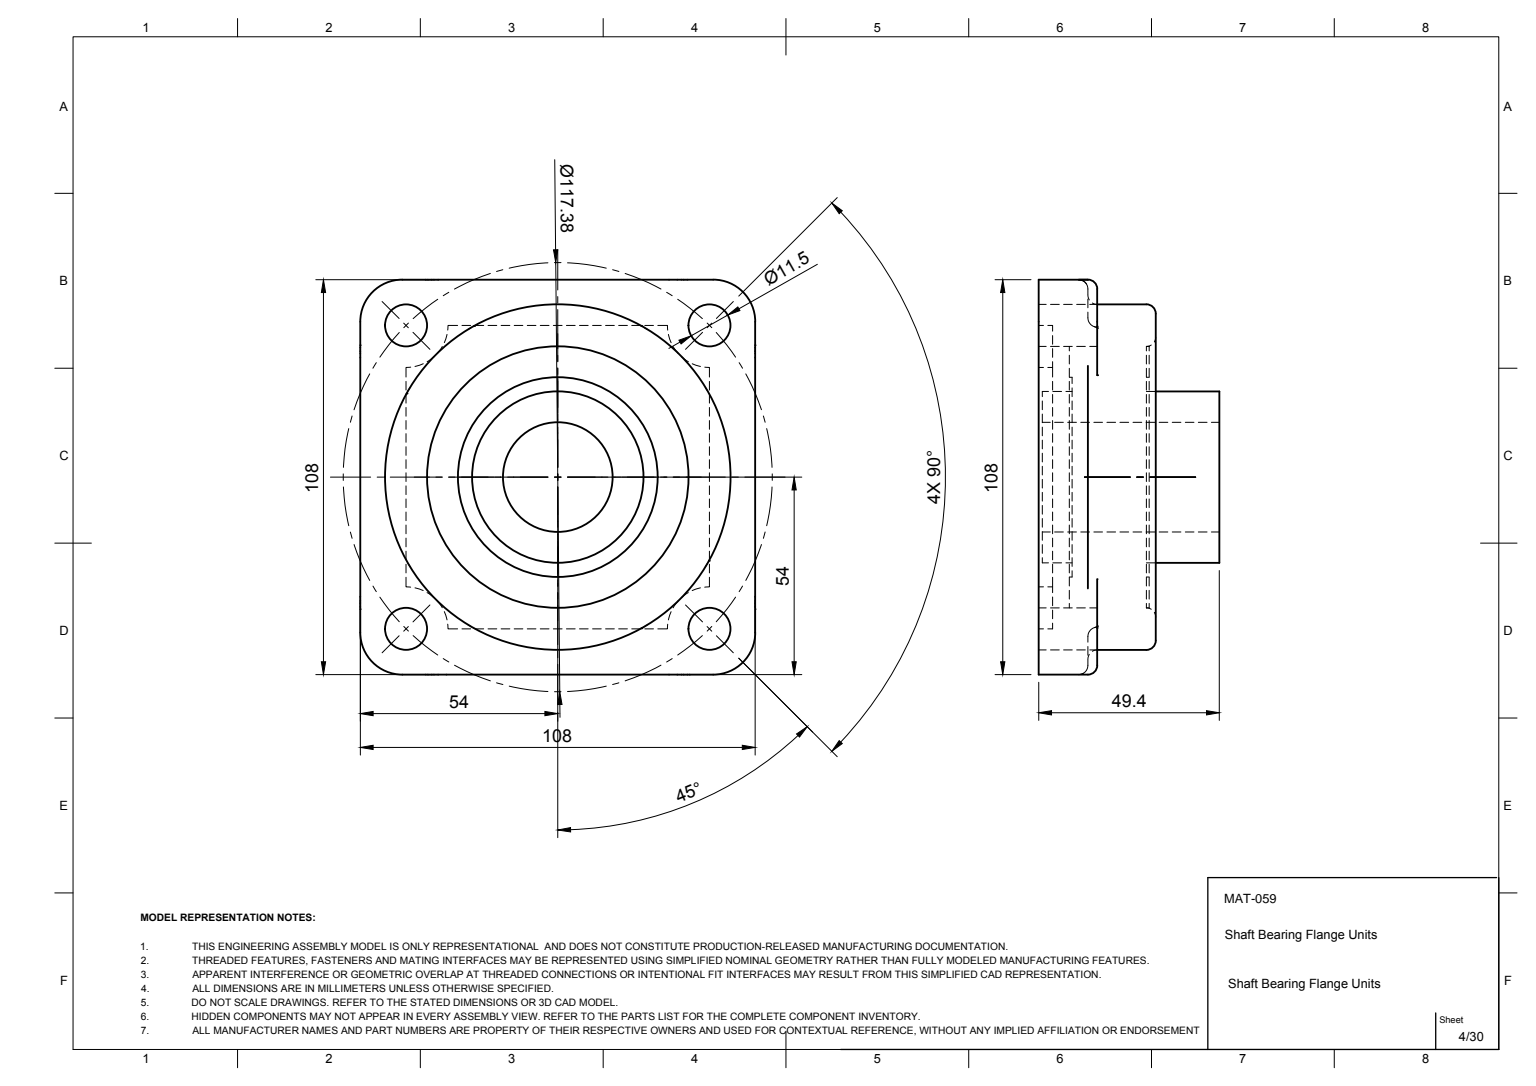
ISO-10303-21;
HEADER;
/* Generated by software containing ST-Developer
 * from STEP Tools, Inc. (www.steptools.com) 
 */

FILE_DESCRIPTION(
/* description */ ('', 'CAx-IF Rec.Pracs.---Representation and Presentation of Product Manufa
cturing Information (PMI)---4.0---2014-10-13'),
/* implementation_level */ '2;1');

FILE_NAME(
/* name */ 'Shaft Bearing Flange Units.step',
/* time_stamp */ '2026-10-28T23:00:48+01:00',
/* author */ (''),
/* organization */ (''),
/* preprocessor_version */ 'ST-DEVELOPER v20.2',
/* originating_system */ 'Autodesk Translation Framework v15.17.0.0',
/* authorisation */ '');

FILE_SCHEMA (('AP242_MANAGED_MODEL_BASED_3D_ENGINEERING_MIM_LF { 1 0 10303 442 2 1 4 }'));
ENDSEC;

DATA;
#10=MECHANICAL_DESIGN_GEOMETRIC_PRESENTATION_REPRESENTATION('',(#962),#61811);
#710=SPHERICAL_SURFACE('',#34223,2.54);
#711=SPHERICAL_SURFACE('',#34226,2.54);
#712=SPHERICAL_SURFACE('',#34247,2.54);
#713=SPHERICAL_SURFACE('',#34253,2.54);
#714=SPHERICAL_SURFACE('',#34261,2.54);
#715=SPHERICAL_SURFACE('',#34268,2.54);
#716=SPHERICAL_SURFACE('',#34273,2.54);
#717=SPHERICAL_SURFACE('',#34278,2.54);
#718=SPHERICAL_SURFACE('',#34289,2.54);
#719=SPHERICAL_SURFACE('',#34304,2.54);
#720=SPHERICAL_SURFACE('',#34315,2.54);
#721=SPHERICAL_SURFACE('',#34321,2.54);
#722=SPHERICAL_SURFACE('',#34322,2.54);
#723=SPHERICAL_SURFACE('',#34332,2.54);
#724=SPHERICAL_SURFACE('',#34340,2.54);
#725=SPHERICAL_SURFACE('',#34343,2.54);
#743=B_SPLINE_CURVE_WITH_KNOTS('',3,(#49121,#49122,#49123,#49124,#49125,
#49126,#49127,#49128,#49129),.UNSPECIFIED.,.F.,.F.,(4,1,1,1,1,1,4),(2.41610505192759E-5,
0.1666666666667,0.3333333333333,0.5,0.6666666666667,0.8333333333333,1.),
 .UNSPECIFIED.);
#744=B_SPLINE_CURVE_WITH_KNOTS('',3,(#49132,#49133,#49134,#49135,#49136,
#49137,#49138,#49139,#49140,#49141,#49142,#49143,#49144,#49145,#49146,#49147,
#49148,#49149,#49150,#49151,#49152,#49153),.UNSPECIFIED.,.F.,.F.,(4,2,2,
2,2,2,2,2,2,2,4),(0.,0.122614489199661,0.166666475605304,0.333332951210507,
0.341573133516598,0.499999426815811,0.560641811243984,0.666665902421115,
0.779351949400631,0.833332378026318,0.999998853631622),.UNSPECIFIED.);
#745=B_SPLINE_CURVE_WITH_KNOTS('',3,(#49162,#49163,#49164,#49165,#49166,
#49167,#49168,#49169,#49170),.UNSPECIFIED.,.F.,.F.,(4,1,1,1,1,1,4),(0.,
0.1666666666667,0.3333333333333,0.5,0.6666666666667,0.8333333333333,1.),
 .UNSPECIFIED.);
#746=B_SPLINE_CURVE_WITH_KNOTS('',3,(#49174,#49175,#49176,#49177,#49178,
#49179,#49180,#49181,#49182),.UNSPECIFIED.,.F.,.F.,(4,1,1,1,1,1,4),(2.85381265954449E-5,
0.1666666666667,0.3333333333333,0.5,0.6666666666667,0.8333333333333,1.),
 .UNSPECIFIED.);
#747=B_SPLINE_CURVE_WITH_KNOTS('',3,(#49186,#49187,#49188,#49189,#49190,
#49191,#49192,#49193,#49194),.UNSPECIFIED.,.F.,.F.,(4,1,1,1,1,1,4),(0.,
0.1666666666667,0.3333333333333,0.5,0.6666666666667,0.8333333333333,1.),
 .UNSPECIFIED.);
#748=B_SPLINE_CURVE_WITH_KNOTS('',3,(#49198,#49199,#49200,#49201,#49202,
#49203,#49204,#49205,#49206),.UNSPECIFIED.,.F.,.F.,(4,1,1,1,1,1,4),(2.416105051936E-5,
0.1666666666667,0.3333333333333,0.5,0.6666666666667,0.8333333333333,1.),
 .UNSPECIFIED.);
#749=B_SPLINE_CURVE_WITH_KNOTS('',3,(#49210,#49211,#49212,#49213,#49214,
#49215,#49216,#49217,#49218),.UNSPECIFIED.,.F.,.F.,(4,1,1,1,1,1,4),(0.,
0.1666666666667,0.3333333333333,0.5,0.6666666666667,0.8333333333333,1.),
 .UNSPECIFIED.);
#750=B_SPLINE_CURVE_WITH_KNOTS('',3,(#49222,#49223,#49224,#49225,#49226,
#49227,#49228,#49229,#49230),.UNSPECIFIED.,.F.,.F.,(4,1,1,1,1,1,4),(2.85380852244383E-5,
0.1666666666667,0.3333333333333,0.5,0.6666666666667,0.8333333333333,1.),
 .UNSPECIFIED.);
#751=B_SPLINE_CURVE_WITH_KNOTS('',3,(#49234,#49235,#49236,#49237,#49238,
#49239,#49240,#49241,#49242),.UNSPECIFIED.,.F.,.F.,(4,1,1,1,1,1,4),(0.,
0.1666666666667,0.3333333333333,0.5,0.6666666666667,0.8333333333333,0.999977439421937),
 .UNSPECIFIED.);
#752=B_SPLINE_CURVE_WITH_KNOTS('',3,(#49287,#49288,#49289,#49290,#49291,
#49292,#49293,#49294,#49295,#49296,#49297,#49298,#49299,#49300,#49301,#49302,
#49303,#49304,#49305,#49306,#49307,#49308,#49309,#49310,#49311,#49312,#49313,
#49314,#49315,#49316,#49317,#49318,#49319,#49320,#49321,#49322,#49323,#49324,
#49325,#49326,#49327,#49328,#49329,#49330,#49331,#49332,#49333,#49334,#49335,
#49336,#49337,#49338,#49339,#49340,#49341),.UNSPECIFIED.,.F.,.F.,(4,3,3,
3,3,3,3,3,3,3,3,3,3,3,3,3,3,3,4),(0.,0.0980466098756701,0.1428571428571,
0.235655762730469,0.2857142857143,0.360443887258383,0.4285714285714,0.5,
0.566042537085864,0.5714285714286,0.636887704333111,0.700301860505849,0.7142857142857,
0.779698786568794,0.844149904052703,0.8571428571429,0.915815433596542,0.97252549736179,
0.999999999993428),.UNSPECIFIED.);
#753=B_SPLINE_CURVE_WITH_KNOTS('',3,(#49366,#49367,#49368,#49369,#49370,
#49371,#49372,#49373,#49374,#49375),.UNSPECIFIED.,.F.,.F.,(4,1,1,1,1,1,
1,4),(0.,0.1428571428571,0.2857142857143,0.4285714285714,0.5714285714286,
0.7142857142857,0.8571428571429,1.),.UNSPECIFIED.);
#754=B_SPLINE_CURVE_WITH_KNOTS('',3,(#49379,#49380,#49381,#49382,#49383,
#49384,#49385,#49386,#49387,#49388),.UNSPECIFIED.,.F.,.F.,(4,1,1,1,1,1,
1,4),(0.,0.1428571428571,0.2857142857143,0.4285714285714,0.5714285714286,
0.7142857142857,0.8571428571429,1.),.UNSPECIFIED.);
#755=B_SPLINE_CURVE_WITH_KNOTS('',3,(#49403,#49404,#49405,#49406,#49407,
#49408,#49409,#49410,#49411,#49412),.UNSPECIFIED.,.F.,.F.,(4,1,1,1,1,1,
1,4),(0.,0.1428571428571,0.2857142857143,0.4285714285714,0.5714285714286,
0.7142857142857,0.8571428571429,1.),.UNSPECIFIED.);
#756=B_SPLINE_CURVE_WITH_KNOTS('',3,(#49415,#49416,#49417,#49418,#49419,
#49420,#49421,#49422,#49423,#49424),.UNSPECIFIED.,.F.,.F.,(4,1,1,1,1,1,
1,4),(0.,0.1428571428571,0.2857142857143,0.4285714285714,0.5714285714286,
0.7142857142857,0.8571428571429,1.),.UNSPECIFIED.);
#757=B_SPLINE_CURVE_WITH_KNOTS('',3,(#49471,#49472,#49473,#49474,#49475,
#49476,#49477,#49478,#49479,#49480,#49481,#49482,#49483,#49484,#49485,#49486,
#49487,#49488,#49489,#49490,#49491,#49492,#49493,#49494,#49495,#49496,#49497,
#49498,#49499,#49500,#49501,#49502,#49503,#49504,#49505,#49506,#49507,#49508,
#49509,#49510,#49511,#49512,#49513,#49514,#49515,#49516,#49517,#49518,#49519,
#49520,#49521,#49522,#49523,#49524,#49525,#49526,#49527,#49528,#49529,#49530,
#49531,#49532,#49533,#49534),.UNSPECIFIED.,.F.,.F.,(4,3,3,3,3,3,3,3,3,3,
3,3,3,3,3,3,3,3,3,3,3,4),(0.,0.022524348752069,0.0826907458045845,0.1428571428571,
0.183969209185199,0.24216625125188,0.2857142857143,0.344939441940217,0.408805968765505,
0.4285714285714,0.494637391748715,0.505902092667849,0.5714285714286,0.644329623937483,
0.666612808947293,0.7142857142857,0.786343515622748,0.827515831049201,0.8571428571429,
0.931638703404591,0.988736971542743,1.),.UNSPECIFIED.);
#758=B_SPLINE_CURVE_WITH_KNOTS('',3,(#49535,#49536,#49537,#49538,#49539,
#49540,#49541,#49542,#49543,#49544,#49545,#49546,#49547,#49548,#49549,#49550,
#49551,#49552,#49553,#49554,#49555,#49556,#49557,#49558,#49559,#49560,#49561,
#49562,#49563,#49564,#49565,#49566,#49567,#49568,#49569,#49570,#49571,#49572,
#49573,#49574,#49575,#49576,#49577),.UNSPECIFIED.,.F.,.F.,(4,3,3,3,3,3,
3,3,3,3,3,3,3,3,4),(0.,0.0708403169631036,0.141196221399192,0.211480985838496,
0.25,0.351421886552124,0.450884598470819,0.5,0.591484098710409,0.684303235352195,
0.75,0.824311643104987,0.900296423629433,0.978409207800814,0.999992340412632),
 .UNSPECIFIED.);
#759=B_SPLINE_CURVE_WITH_KNOTS('',3,(#49622,#49623,#49624,#49625,#49626,
#49627,#49628,#49629,#49630,#49631,#49632,#49633,#49634,#49635,#49636,#49637,
#49638,#49639,#49640,#49641,#49642,#49643),.UNSPECIFIED.,.F.,.F.,(4,2,2,
2,2,2,2,2,2,2,4),(1.17968190133454E-6,0.166667646133106,0.219922777256081,
0.333334116906424,0.439180276291458,0.500000587679843,0.658731994343029,
0.666667058453262,0.833333529226581,0.87820409141329,1.),.UNSPECIFIED.);
#760=B_SPLINE_CURVE_WITH_KNOTS('',3,(#49690,#49691,#49692,#49693,#49694,
#49695,#49696,#49697,#49698),.UNSPECIFIED.,.F.,.F.,(4,1,1,1,1,1,4),(0.,
0.1666666666667,0.3333333333333,0.5,0.6666666666667,0.8333333333333,0.999998808810884),
 .UNSPECIFIED.);
#761=B_SPLINE_CURVE_WITH_KNOTS('',3,(#49749,#49750,#49751,#49752,#49753,
#49754,#49755,#49756,#49757,#49758,#49759,#49760,#49761,#49762,#49763,#49764,
#49765,#49766,#49767,#49768,#49769,#49770,#49771,#49772,#49773,#49774,#49775,
#49776,#49777,#49778,#49779,#49780,#49781,#49782,#49783,#49784,#49785,#49786,
#49787,#49788,#49789,#49790,#49791,#49792,#49793,#49794,#49795,#49796,#49797,
#49798,#49799,#49800,#49801,#49802,#49803,#49804,#49805,#49806,#49807,#49808,
#49809,#49810,#49811,#49812),.UNSPECIFIED.,.F.,.F.,(4,3,3,3,3,3,3,3,3,3,
3,3,3,3,3,3,3,3,3,3,3,4),(0.,0.011263028288939,0.0857588259046287,0.1428571428571,
0.172484168893865,0.244542016262902,0.2857142857143,0.33338719123398,0.406288255376173,
0.4285714285714,0.49409790740126,0.560163866020983,0.5714285714286,0.635295097422919,
0.655060558117981,0.7142857142857,0.77248275702656,0.81603079085385,0.8571428571429,
0.917309254199729,0.977475651256559,1.),.UNSPECIFIED.);
#762=B_SPLINE_CURVE_WITH_KNOTS('',3,(#49861,#49862,#49863,#49864,#49865,
#49866,#49867,#49868,#49869,#49870,#49871,#49872,#49873,#49874,#49875,#49876,
#49877,#49878,#49879,#49880,#49881,#49882,#49883,#49884,#49885,#49886,#49887,
#49888,#49889,#49890,#49891,#49892,#49893,#49894,#49895,#49896,#49897,#49898,
#49899,#49900,#49901,#49902,#49903,#49904,#49905,#49906,#49907,#49908,#49909,
#49910,#49911,#49912,#49913,#49914,#49915,#49916,#49917,#49918,#49919,#49920,
#49921,#49922,#49923,#49924),.UNSPECIFIED.,.F.,.F.,(4,3,3,3,3,3,3,3,3,3,
3,3,3,3,3,3,3,3,3,3,3,4),(0.,0.022524348752069,0.0826907458045845,0.1428571428571,
0.183969209185192,0.242166251253732,0.2857142857143,0.34493944194013,0.408805968765661,
0.4285714285714,0.494637391744036,0.505902092667695,0.5714285714286,0.644329623939086,
0.666612808947312,0.7142857142857,0.786343515622548,0.827515831048836,0.8571428571429,
0.931638703405425,0.988736971542787,1.),.UNSPECIFIED.);
#763=B_SPLINE_CURVE_WITH_KNOTS('',3,(#49925,#49926,#49927,#49928,#49929,
#49930,#49931,#49932,#49933,#49934,#49935,#49936,#49937,#49938,#49939,#49940,
#49941,#49942,#49943,#49944,#49945,#49946,#49947,#49948,#49949,#49950,#49951,
#49952,#49953,#49954,#49955,#49956,#49957,#49958,#49959,#49960,#49961,#49962,
#49963,#49964,#49965,#49966,#49967),.UNSPECIFIED.,.F.,.F.,(4,3,3,3,3,3,
3,3,3,3,3,3,3,3,4),(0.,0.0708403169625752,0.141196221398188,0.211480985837894,
0.25,0.351421886557641,0.45088459847787,0.5,0.591484098711512,0.684303235350053,
0.75,0.824311643104386,0.900296423628743,0.978409207797605,0.999992340412643),
 .UNSPECIFIED.);
#764=B_SPLINE_CURVE_WITH_KNOTS('',3,(#50011,#50012,#50013,#50014,#50015,
#50016,#50017,#50018,#50019),.UNSPECIFIED.,.F.,.F.,(4,1,1,1,1,1,4),(1.12301924736311E-6,
0.1666666666667,0.3333333333333,0.5,0.6666666666667,0.8333333333333,1.),
 .UNSPECIFIED.);
#765=B_SPLINE_CURVE_WITH_KNOTS('',3,(#50069,#50070,#50071,#50072,#50073,
#50074,#50075,#50076,#50077,#50078,#50079,#50080,#50081,#50082,#50083,#50084,
#50085,#50086,#50087,#50088,#50089,#50090),.UNSPECIFIED.,.F.,.F.,(4,2,2,
2,2,2,2,2,2,2,4),(1.17968190350786E-6,0.166667646133105,0.219922777256189,
0.333334116906424,0.439180276291488,0.500000587679843,0.658731994343154,
0.666667058453262,0.833333529226581,0.878204091413217,1.),.UNSPECIFIED.);
#766=B_SPLINE_CURVE_WITH_KNOTS('',3,(#50099,#50100,#50101,#50102,#50103,
#50104,#50105,#50106,#50107,#50108,#50109,#50110,#50111,#50112,#50113,#50114,
#50115,#50116,#50117,#50118,#50119,#50120,#50121,#50122,#50123,#50124,#50125,
#50126,#50127,#50128,#50129,#50130,#50131,#50132,#50133,#50134,#50135,#50136,
#50137,#50138,#50139,#50140,#50141,#50142,#50143,#50144,#50145,#50146,#50147,
#50148,#50149,#50150,#50151,#50152,#50153),.UNSPECIFIED.,.F.,.F.,(4,3,3,
3,3,3,3,3,3,3,3,3,3,3,3,3,3,3,4),(0.,0.0565152922712344,0.114965932003303,
0.1428571428571,0.207266907155971,0.272629548288784,0.2857142857143,0.349038397788053,
0.414377828143602,0.4285714285714,0.494613972575815,0.562439737569692,0.5714285714286,
0.646158146057277,0.7142857142857,0.807084236549117,0.8571428571429,0.955189540194312,
1.),.UNSPECIFIED.);
#767=B_SPLINE_CURVE_WITH_KNOTS('',3,(#50200,#50201,#50202,#50203,#50204,
#50205,#50206,#50207,#50208,#50209,#50210,#50211,#50212,#50213,#50214,#50215,
#50216,#50217,#50218,#50219,#50220,#50221,#50222,#50223,#50224,#50225,#50226,
#50227,#50228,#50229,#50230,#50231,#50232,#50233,#50234,#50235,#50236,#50237,
#50238,#50239,#50240,#50241,#50242),.UNSPECIFIED.,.F.,.F.,(4,3,3,3,3,3,
3,3,3,3,3,3,3,3,4),(0.,0.0708403169627012,0.141196221397882,0.211480985835855,
0.25,0.351421886559069,0.450884598479571,0.5,0.591484098710457,0.684303235349992,
0.75,0.824311643105781,0.900296423630328,0.97840920780083,0.999992340411847),
 .UNSPECIFIED.);
#768=B_SPLINE_CURVE_WITH_KNOTS('',3,(#50244,#50245,#50246,#50247,#50248,
#50249,#50250,#50251,#50252,#50253),.UNSPECIFIED.,.F.,.F.,(4,1,1,1,1,1,
1,4),(0.,0.1428571428571,0.2857142857143,0.4285714285714,0.5714285714286,
0.7142857142857,0.8571428571429,1.),.UNSPECIFIED.);
#769=B_SPLINE_CURVE_WITH_KNOTS('',3,(#50260,#50261,#50262,#50263,#50264,
#50265,#50266,#50267,#50268,#50269),.UNSPECIFIED.,.F.,.F.,(4,1,1,1,1,1,
1,4),(0.,0.1428571428571,0.2857142857143,0.4285714285714,0.5714285714286,
0.7142857142857,0.8571428571429,1.),.UNSPECIFIED.);
#770=B_SPLINE_CURVE_WITH_KNOTS('',3,(#50286,#50287,#50288,#50289,#50290,
#50291,#50292,#50293,#50294,#50295),.UNSPECIFIED.,.F.,.F.,(4,1,1,1,1,1,
1,4),(0.,0.1428571428571,0.2857142857143,0.4285714285714,0.5714285714286,
0.7142857142857,0.8571428571429,1.),.UNSPECIFIED.);
#771=B_SPLINE_CURVE_WITH_KNOTS('',3,(#50299,#50300,#50301,#50302,#50303,
#50304,#50305,#50306,#50307,#50308),.UNSPECIFIED.,.F.,.F.,(4,1,1,1,1,1,
1,4),(0.,0.1428571428571,0.2857142857143,0.4285714285714,0.5714285714286,
0.7142857142857,0.8571428571429,1.),.UNSPECIFIED.);
#772=B_SPLINE_CURVE_WITH_KNOTS('',3,(#50318,#50319,#50320,#50321,#50322,
#50323,#50324,#50325,#50326),.UNSPECIFIED.,.F.,.F.,(4,1,1,1,1,1,4),(1.1230192517404E-6,
0.1666666666667,0.3333333333333,0.5,0.6666666666667,0.8333333333333,1.),
 .UNSPECIFIED.);
#773=B_SPLINE_CURVE_WITH_KNOTS('',3,(#50406,#50407,#50408,#50409,#50410,
#50411,#50412,#50413,#50414,#50415,#50416,#50417,#50418,#50419,#50420,#50421,
#50422,#50423,#50424,#50425,#50426,#50427),.UNSPECIFIED.,.F.,.F.,(4,2,2,
2,2,2,2,2,2,2,4),(0.,0.122614489199695,0.166666475605304,0.333332951210509,
0.341573133516643,0.499999426815813,0.560641811244011,0.666665902421118,
0.779351949400641,0.833332378026322,0.999998853631626),.UNSPECIFIED.);
#774=B_SPLINE_CURVE_WITH_KNOTS('',3,(#50478,#50479,#50480,#50481,#50482,
#50483,#50484,#50485,#50486,#50487,#50488,#50489,#50490,#50491,#50492,#50493,
#50494,#50495,#50496,#50497,#50498,#50499,#50500,#50501,#50502,#50503,#50504,
#50505,#50506,#50507,#50508,#50509,#50510,#50511,#50512,#50513,#50514,#50515,
#50516,#50517,#50518,#50519,#50520,#50521,#50522,#50523,#50524,#50525,#50526,
#50527,#50528,#50529,#50530,#50531,#50532,#50533,#50534,#50535,#50536,#50537,
#50538,#50539,#50540,#50541),.UNSPECIFIED.,.F.,.F.,(4,3,3,3,3,3,3,3,3,3,
3,3,3,3,3,3,3,3,3,3,3,4),(0.,0.0112630282889006,0.0857588259025268,0.142857142855473,
0.172484168891931,0.244542016261801,0.285714285711046,0.333387191230076,
0.406288255372341,0.428571428566519,0.49409790739575,0.560163866013515,
0.571428571422092,0.635295097422519,0.655060558110842,0.714285714277565,
0.772482757008491,0.816030790845477,0.857142857133138,0.917309254189421,
0.977475651245705,0.999999999988612),.UNSPECIFIED.);
#775=B_SPLINE_CURVE_WITH_KNOTS('',3,(#50551,#50552,#50553,#50554,#50555,
#50556,#50557,#50558,#50559,#50560,#50561,#50562,#50563,#50564,#50565,#50566,
#50567,#50568,#50569,#50570,#50571,#50572,#50573,#50574,#50575,#50576,#50577,
#50578,#50579,#50580,#50581,#50582,#50583,#50584,#50585,#50586,#50587,#50588,
#50589,#50590,#50591,#50592,#50593,#50594,#50595,#50596,#50597,#50598,#50599,
#50600,#50601,#50602,#50603,#50604,#50605),.UNSPECIFIED.,.F.,.F.,(4,3,3,
3,3,3,3,3,3,3,3,3,3,3,3,3,3,3,4),(0.,0.0565152922717072,0.114965932004273,
0.1428571428571,0.207266907154939,0.272629548286749,0.2857142857143,0.349038397790888,
0.414377828149668,0.4285714285714,0.494613972566219,0.562439737549771,0.5714285714286,
0.64615814615571,0.7142857142857,0.807084237689468,0.8571428571429,0.955189538087307,
1.),.UNSPECIFIED.);
#776=B_SPLINE_CURVE_WITH_KNOTS('',3,(#50699,#50700,#50701,#50702,#50703,
#50704,#50705,#50706,#50707,#50708,#50709,#50710,#50711,#50712,#50713,#50714,
#50715,#50716,#50717,#50718,#50719,#50720,#50721,#50722,#50723,#50724,#50725,
#50726,#50727,#50728,#50729,#50730,#50731,#50732,#50733,#50734,#50735,#50736,
#50737,#50738,#50739,#50740,#50741,#50742,#50743,#50744,#50745,#50746,#50747,
#50748,#50749,#50750,#50751,#50752,#50753,#50754,#50755,#50756,#50757,#50758,
#50759,#50760,#50761,#50762),.UNSPECIFIED.,.F.,.F.,(4,3,3,3,3,3,3,3,3,3,
3,3,3,3,3,3,3,3,3,3,3,4),(0.,0.011263028289029,0.0857588259024072,0.1428571428571,
0.172484168893897,0.244542016269632,0.2857142857143,0.333387191233873,0.406288255371836,
0.4285714285714,0.494097907401377,0.560163866020033,0.5714285714286,0.63529509742806,
0.655060558118314,0.7142857142857,0.772482757018248,0.816030790854834,0.8571428571429,
0.917309254199805,0.97747565125671,0.999999999999998),.UNSPECIFIED.);
#777=B_SPLINE_CURVE_WITH_KNOTS('',3,(#50807,#50808,#50809,#50810,#50811,
#50812,#50813,#50814,#50815),.UNSPECIFIED.,.F.,.F.,(4,1,1,1,1,1,4),(0.,
0.1666666666667,0.3333333333333,0.5,0.6666666666667,0.8333333333333,0.999998808810887),
 .UNSPECIFIED.);
#854=(
BOUNDED_SURFACE()
B_SPLINE_SURFACE(3,3,((#49084,#49085,#49086,#49087,#49088,#49089,#49090,
#49091,#49092),(#49093,#49094,#49095,#49096,#49097,#49098,#49099,#49100,
#49101),(#49102,#49103,#49104,#49105,#49106,#49107,#49108,#49109,#49110),
(#49111,#49112,#49113,#49114,#49115,#49116,#49117,#49118,#49119)),
 .UNSPECIFIED.,.F.,.F.,.F.)
B_SPLINE_SURFACE_WITH_KNOTS((4,4),(4,1,1,1,1,1,4),(0.,1.),(0.1657185475802,
0.2191677809649,0.2917200555518,0.3628106421009,0.4321191894168,0.5006571708278,
0.5134509073716),.UNSPECIFIED.)
GEOMETRIC_REPRESENTATION_ITEM()
RATIONAL_B_SPLINE_SURFACE(((1.212997002425,1.212997002425,1.212997002425,
1.212997002425,1.212997002425,1.212997002425,1.212997002425,1.212997002425,
1.212997002425),(0.9290009991916,0.9290009991916,0.9290009991916,0.9290009991916,
0.9290009991916,0.9290009991916,0.9290009991916,0.9290009991916,0.9290009991916),
(0.9290009991916,0.9290009991916,0.9290009991916,0.9290009991916,0.9290009991916,
0.9290009991916,0.9290009991916,0.9290009991916,0.9290009991916),(1.212997002425,
1.212997002425,1.212997002425,1.212997002425,1.212997002425,1.212997002425,
1.212997002425,1.212997002425,1.212997002425)))
REPRESENTATION_ITEM('')
SURFACE()
);
#855=(
BOUNDED_SURFACE()
B_SPLINE_SURFACE(3,3,((#49426,#49427,#49428,#49429,#49430,#49431,#49432,
#49433,#49434,#49435,#49436),(#49437,#49438,#49439,#49440,#49441,#49442,
#49443,#49444,#49445,#49446,#49447),(#49448,#49449,#49450,#49451,#49452,
#49453,#49454,#49455,#49456,#49457,#49458),(#49459,#49460,#49461,#49462,
#49463,#49464,#49465,#49466,#49467,#49468,#49469)),.UNSPECIFIED.,.F.,.F.,
 .F.)
B_SPLINE_SURFACE_WITH_KNOTS((4,4),(4,1,1,1,1,1,1,1,4),(0.,1.),(0.4912064856134,
0.5104451093027,0.5824328871872,0.6465099292207,0.7028608084679,0.7531387245364,
0.7991472729598,0.8414732732765,0.8528970245468),.UNSPECIFIED.)
GEOMETRIC_REPRESENTATION_ITEM()
RATIONAL_B_SPLINE_SURFACE(((1.212994991089,1.212994991089,1.212994991089,
1.212994991089,1.212994991089,1.212994991089,1.212994991089,1.212994991089,
1.212994991089,1.212994991089,1.212994991089),(0.9290016696369,0.9290016696369,
0.9290016696369,0.9290016696369,0.9290016696369,0.9290016696369,0.9290016696369,
0.9290016696369,0.9290016696369,0.9290016696369,0.9290016696369),(0.9290016696369,
0.9290016696369,0.9290016696369,0.9290016696369,0.9290016696369,0.9290016696369,
0.9290016696369,0.9290016696369,0.9290016696369,0.9290016696369,0.9290016696369),
(1.212994991089,1.212994991089,1.212994991089,1.212994991089,1.212994991089,
1.212994991089,1.212994991089,1.212994991089,1.212994991089,1.212994991089,
1.212994991089)))
REPRESENTATION_ITEM('')
SURFACE()
);
#856=(
BOUNDED_SURFACE()
B_SPLINE_SURFACE(3,3,((#49586,#49587,#49588,#49589,#49590,#49591,#49592,
#49593,#49594),(#49595,#49596,#49597,#49598,#49599,#49600,#49601,#49602,
#49603),(#49604,#49605,#49606,#49607,#49608,#49609,#49610,#49611,#49612),
(#49613,#49614,#49615,#49616,#49617,#49618,#49619,#49620,#49621)),
 .UNSPECIFIED.,.F.,.F.,.F.)
B_SPLINE_SURFACE_WITH_KNOTS((4,4),(4,1,1,1,1,1,4),(0.,1.),(0.4865185456842,
0.4989653295554,0.5676881330315,0.6372726174693,0.7085358956321,0.7811839361635,
0.8342456994508),.UNSPECIFIED.)
GEOMETRIC_REPRESENTATION_ITEM()
RATIONAL_B_SPLINE_SURFACE(((1.212997004616,1.212997004616,1.212997004616,
1.212997004616,1.212997004616,1.212997004616,1.212997004616,1.212997004616,
1.212997004616),(0.9290009984612,0.9290009984612,0.9290009984612,0.9290009984612,
0.9290009984612,0.9290009984612,0.9290009984612,0.9290009984612,0.9290009984612),
(0.9290009984612,0.9290009984612,0.9290009984612,0.9290009984612,0.9290009984612,
0.9290009984612,0.9290009984612,0.9290009984612,0.9290009984612),(1.212997004616,
1.212997004616,1.212997004616,1.212997004616,1.212997004616,1.212997004616,
1.212997004616,1.212997004616,1.212997004616)))
REPRESENTATION_ITEM('')
SURFACE()
);
#857=(
BOUNDED_SURFACE()
B_SPLINE_SURFACE(3,3,((#49652,#49653,#49654,#49655,#49656,#49657,#49658,
#49659,#49660),(#49661,#49662,#49663,#49664,#49665,#49666,#49667,#49668,
#49669),(#49670,#49671,#49672,#49673,#49674,#49675,#49676,#49677,#49678),
(#49679,#49680,#49681,#49682,#49683,#49684,#49685,#49686,#49687)),
 .UNSPECIFIED.,.F.,.F.,.F.)
B_SPLINE_SURFACE_WITH_KNOTS((4,4),(4,1,1,1,1,1,4),(0.,1.),(0.1657200365356,
0.218898549315,0.2912491980129,0.3619657900993,0.4315535161345,0.500650977664,
0.5134507157886),.UNSPECIFIED.)
GEOMETRIC_REPRESENTATION_ITEM()
RATIONAL_B_SPLINE_SURFACE(((1.212996916314,1.212996916314,1.212996916314,
1.212996916314,1.212996916314,1.212996916314,1.212996916314,1.212996916314,
1.212996916314),(0.9290010278954,0.9290010278954,0.9290010278954,0.9290010278954,
0.9290010278954,0.9290010278954,0.9290010278954,0.9290010278954,0.9290010278954),
(0.9290010278954,0.9290010278954,0.9290010278954,0.9290010278954,0.9290010278954,
0.9290010278954,0.9290010278954,0.9290010278954,0.9290010278954),(1.212996916314,
1.212996916314,1.212996916314,1.212996916314,1.212996916314,1.212996916314,
1.212996916314,1.212996916314,1.212996916314)))
REPRESENTATION_ITEM('')
SURFACE()
);
#858=(
BOUNDED_SURFACE()
B_SPLINE_SURFACE(3,3,((#49705,#49706,#49707,#49708,#49709,#49710,#49711,
#49712,#49713,#49714,#49715),(#49716,#49717,#49718,#49719,#49720,#49721,
#49722,#49723,#49724,#49725,#49726),(#49727,#49728,#49729,#49730,#49731,
#49732,#49733,#49734,#49735,#49736,#49737),(#49738,#49739,#49740,#49741,
#49742,#49743,#49744,#49745,#49746,#49747,#49748)),.UNSPECIFIED.,.F.,.F.,
 .F.)
B_SPLINE_SURFACE_WITH_KNOTS((4,4),(4,1,1,1,1,1,1,1,4),(0.,1.),(0.1471313081811,
0.1585267267235,0.2008527270402,0.2468612754635,0.297139191532,0.3534900707792,
0.4175671128126,0.4895548906971,0.5087566656269),.UNSPECIFIED.)
GEOMETRIC_REPRESENTATION_ITEM()
RATIONAL_B_SPLINE_SURFACE(((1.212994990549,1.212994990549,1.212994990549,
1.212994990549,1.212994990549,1.212994990549,1.212994990549,1.212994990549,
1.212994990549,1.212994990549,1.212994990549),(0.9290016698171,0.9290016698171,
0.9290016698171,0.9290016698171,0.9290016698171,0.9290016698171,0.9290016698171,
0.9290016698171,0.9290016698171,0.9290016698171,0.9290016698171),(0.9290016698171,
0.9290016698171,0.9290016698171,0.9290016698171,0.9290016698171,0.9290016698171,
0.9290016698171,0.9290016698171,0.9290016698171,0.9290016698171,0.9290016698171),
(1.212994990549,1.212994990549,1.212994990549,1.212994990549,1.212994990549,
1.212994990549,1.212994990549,1.212994990549,1.212994990549,1.212994990549,
1.212994990549)))
REPRESENTATION_ITEM('')
SURFACE()
);
#859=(
BOUNDED_SURFACE()
B_SPLINE_SURFACE(3,3,((#49816,#49817,#49818,#49819,#49820,#49821,#49822,
#49823,#49824,#49825,#49826),(#49827,#49828,#49829,#49830,#49831,#49832,
#49833,#49834,#49835,#49836,#49837),(#49838,#49839,#49840,#49841,#49842,
#49843,#49844,#49845,#49846,#49847,#49848),(#49849,#49850,#49851,#49852,
#49853,#49854,#49855,#49856,#49857,#49858,#49859)),.UNSPECIFIED.,.F.,.F.,
 .F.)
B_SPLINE_SURFACE_WITH_KNOTS((4,4),(4,1,1,1,1,1,1,1,4),(0.,1.),(0.4912064856134,
0.5104451093027,0.5824328871872,0.6465099292207,0.7028608084679,0.7531387245364,
0.7991472729597,0.8414732732765,0.8528970245468),.UNSPECIFIED.)
GEOMETRIC_REPRESENTATION_ITEM()
RATIONAL_B_SPLINE_SURFACE(((1.212994991089,1.212994991089,1.212994991089,
1.212994991089,1.212994991089,1.212994991089,1.212994991089,1.212994991089,
1.212994991089,1.212994991089,1.212994991089),(0.9290016696369,0.9290016696369,
0.9290016696369,0.9290016696369,0.9290016696369,0.9290016696369,0.9290016696369,
0.9290016696369,0.9290016696369,0.9290016696369,0.9290016696369),(0.9290016696369,
0.9290016696369,0.9290016696369,0.9290016696369,0.9290016696369,0.9290016696369,
0.9290016696369,0.9290016696369,0.9290016696369,0.9290016696369,0.9290016696369),
(1.212994991089,1.212994991089,1.212994991089,1.212994991089,1.212994991089,
1.212994991089,1.212994991089,1.212994991089,1.212994991089,1.212994991089,
1.212994991089)))
REPRESENTATION_ITEM('')
SURFACE()
);
#860=(
BOUNDED_SURFACE()
B_SPLINE_SURFACE(3,3,((#49975,#49976,#49977,#49978,#49979,#49980,#49981,
#49982,#49983),(#49984,#49985,#49986,#49987,#49988,#49989,#49990,#49991,
#49992),(#49993,#49994,#49995,#49996,#49997,#49998,#49999,#50000,#50001),
(#50002,#50003,#50004,#50005,#50006,#50007,#50008,#50009,#50010)),
 .UNSPECIFIED.,.F.,.F.,.F.)
B_SPLINE_SURFACE_WITH_KNOTS((4,4),(4,1,1,1,1,1,4),(0.,1.),(0.4865169701774,
0.499349022336,0.5684464838655,0.6380342099007,0.7087508019872,0.781101450685,
0.8342465447531),.UNSPECIFIED.)
GEOMETRIC_REPRESENTATION_ITEM()
RATIONAL_B_SPLINE_SURFACE(((1.21299691379,1.21299691379,1.21299691379,1.21299691379,
1.21299691379,1.21299691379,1.21299691379,1.21299691379,1.21299691379),
(0.9290010287368,0.9290010287368,0.9290010287368,0.9290010287368,0.9290010287368,
0.9290010287368,0.9290010287368,0.9290010287368,0.9290010287368),(0.9290010287368,
0.9290010287368,0.9290010287368,0.9290010287368,0.9290010287368,0.9290010287368,
0.9290010287368,0.9290010287368,0.9290010287368),(1.21299691379,1.21299691379,
1.21299691379,1.21299691379,1.21299691379,1.21299691379,1.21299691379,1.21299691379,
1.21299691379)))
REPRESENTATION_ITEM('')
SURFACE()
);
#861=(
BOUNDED_SURFACE()
B_SPLINE_SURFACE(3,3,((#50032,#50033,#50034,#50035,#50036,#50037,#50038,
#50039,#50040),(#50041,#50042,#50043,#50044,#50045,#50046,#50047,#50048,
#50049),(#50050,#50051,#50052,#50053,#50054,#50055,#50056,#50057,#50058),
(#50059,#50060,#50061,#50062,#50063,#50064,#50065,#50066,#50067)),
 .UNSPECIFIED.,.F.,.F.,.F.)
B_SPLINE_SURFACE_WITH_KNOTS((4,4),(4,1,1,1,1,1,4),(0.,1.),(0.4865185456842,
0.4989653295554,0.5676881330316,0.6372726174694,0.7085358956322,0.7811839361635,
0.8342456994508),.UNSPECIFIED.)
GEOMETRIC_REPRESENTATION_ITEM()
RATIONAL_B_SPLINE_SURFACE(((1.212997004616,1.212997004616,1.212997004616,
1.212997004616,1.212997004616,1.212997004616,1.212997004616,1.212997004616,
1.212997004616),(0.9290009984612,0.9290009984612,0.9290009984612,0.9290009984612,
0.9290009984612,0.9290009984612,0.9290009984612,0.9290009984612,0.9290009984612),
(0.9290009984612,0.9290009984612,0.9290009984612,0.9290009984612,0.9290009984612,
0.9290009984612,0.9290009984612,0.9290009984612,0.9290009984612),(1.212997004616,
1.212997004616,1.212997004616,1.212997004616,1.212997004616,1.212997004616,
1.212997004616,1.212997004616,1.212997004616)))
REPRESENTATION_ITEM('')
SURFACE()
);
#862=(
BOUNDED_SURFACE()
B_SPLINE_SURFACE(3,3,((#50155,#50156,#50157,#50158,#50159,#50160,#50161,
#50162,#50163,#50164,#50165),(#50166,#50167,#50168,#50169,#50170,#50171,
#50172,#50173,#50174,#50175,#50176),(#50177,#50178,#50179,#50180,#50181,
#50182,#50183,#50184,#50185,#50186,#50187),(#50188,#50189,#50190,#50191,
#50192,#50193,#50194,#50195,#50196,#50197,#50198)),.UNSPECIFIED.,.F.,.F.,
 .F.)
B_SPLINE_SURFACE_WITH_KNOTS((4,4),(4,1,1,1,1,1,1,1,4),(0.,1.),(0.4912064856134,
0.5104451093027,0.5824328871873,0.6465099292207,0.7028608084679,0.7531387245365,
0.7991472729598,0.8414732732765,0.8528970245468),.UNSPECIFIED.)
GEOMETRIC_REPRESENTATION_ITEM()
RATIONAL_B_SPLINE_SURFACE(((1.212994991089,1.212994991089,1.212994991089,
1.212994991089,1.212994991089,1.212994991089,1.212994991089,1.212994991089,
1.212994991089,1.212994991089,1.212994991089),(0.9290016696369,0.9290016696369,
0.9290016696369,0.9290016696369,0.9290016696369,0.9290016696369,0.9290016696369,
0.9290016696369,0.9290016696369,0.9290016696369,0.9290016696369),(0.9290016696369,
0.9290016696369,0.9290016696369,0.9290016696369,0.9290016696369,0.9290016696369,
0.9290016696369,0.9290016696369,0.9290016696369,0.9290016696369,0.9290016696369),
(1.212994991089,1.212994991089,1.212994991089,1.212994991089,1.212994991089,
1.212994991089,1.212994991089,1.212994991089,1.212994991089,1.212994991089,
1.212994991089)))
REPRESENTATION_ITEM('')
SURFACE()
);
#863=(
BOUNDED_SURFACE()
B_SPLINE_SURFACE(3,3,((#50328,#50329,#50330,#50331,#50332,#50333,#50334,
#50335,#50336),(#50337,#50338,#50339,#50340,#50341,#50342,#50343,#50344,
#50345),(#50346,#50347,#50348,#50349,#50350,#50351,#50352,#50353,#50354),
(#50355,#50356,#50357,#50358,#50359,#50360,#50361,#50362,#50363)),
 .UNSPECIFIED.,.F.,.F.,.F.)
B_SPLINE_SURFACE_WITH_KNOTS((4,4),(4,1,1,1,1,1,4),(0.,1.),(0.4865169701774,
0.499349022336,0.5684464838655,0.6380342099007,0.7087508019872,0.781101450685,
0.8342465447531),.UNSPECIFIED.)
GEOMETRIC_REPRESENTATION_ITEM()
RATIONAL_B_SPLINE_SURFACE(((1.21299691379,1.21299691379,1.21299691379,1.21299691379,
1.21299691379,1.21299691379,1.21299691379,1.21299691379,1.21299691379),
(0.9290010287368,0.9290010287368,0.9290010287368,0.9290010287368,0.9290010287368,
0.9290010287368,0.9290010287368,0.9290010287368,0.9290010287368),(0.9290010287368,
0.9290010287368,0.9290010287368,0.9290010287368,0.9290010287368,0.9290010287368,
0.9290010287368,0.9290010287368,0.9290010287368),(1.21299691379,1.21299691379,
1.21299691379,1.21299691379,1.21299691379,1.21299691379,1.21299691379,1.21299691379,
1.21299691379)))
REPRESENTATION_ITEM('')
SURFACE()
);
#864=(
BOUNDED_SURFACE()
B_SPLINE_SURFACE(3,3,((#50368,#50369,#50370,#50371,#50372,#50373,#50374,
#50375,#50376),(#50377,#50378,#50379,#50380,#50381,#50382,#50383,#50384,
#50385),(#50386,#50387,#50388,#50389,#50390,#50391,#50392,#50393,#50394),
(#50395,#50396,#50397,#50398,#50399,#50400,#50401,#50402,#50403)),
 .UNSPECIFIED.,.F.,.F.,.F.)
B_SPLINE_SURFACE_WITH_KNOTS((4,4),(4,1,1,1,1,1,4),(0.,1.),(0.1657185475802,
0.2191677809649,0.2917200555518,0.3628106421009,0.4321191894168,0.5006571708278,
0.5134509073716),.UNSPECIFIED.)
GEOMETRIC_REPRESENTATION_ITEM()
RATIONAL_B_SPLINE_SURFACE(((1.212997002425,1.212997002425,1.212997002425,
1.212997002425,1.212997002425,1.212997002425,1.212997002425,1.212997002425,
1.212997002425),(0.9290009991916,0.9290009991916,0.9290009991916,0.9290009991916,
0.9290009991916,0.9290009991916,0.9290009991916,0.9290009991916,0.9290009991916),
(0.9290009991916,0.9290009991916,0.9290009991916,0.9290009991916,0.9290009991916,
0.9290009991916,0.9290009991916,0.9290009991916,0.9290009991916),(1.212997002425,
1.212997002425,1.212997002425,1.212997002425,1.212997002425,1.212997002425,
1.212997002425,1.212997002425,1.212997002425)))
REPRESENTATION_ITEM('')
SURFACE()
);
#865=(
BOUNDED_SURFACE()
B_SPLINE_SURFACE(3,3,((#50434,#50435,#50436,#50437,#50438,#50439,#50440,
#50441,#50442,#50443,#50444),(#50445,#50446,#50447,#50448,#50449,#50450,
#50451,#50452,#50453,#50454,#50455),(#50456,#50457,#50458,#50459,#50460,
#50461,#50462,#50463,#50464,#50465,#50466),(#50467,#50468,#50469,#50470,
#50471,#50472,#50473,#50474,#50475,#50476,#50477)),.UNSPECIFIED.,.F.,.F.,
 .F.)
B_SPLINE_SURFACE_WITH_KNOTS((4,4),(4,1,1,1,1,1,1,1,4),(0.,1.),(0.1471313081811,
0.1585267267235,0.2008527270402,0.2468612754635,0.2971391915321,0.3534900707793,
0.4175671128127,0.4895548906973,0.5087566656269),.UNSPECIFIED.)
GEOMETRIC_REPRESENTATION_ITEM()
RATIONAL_B_SPLINE_SURFACE(((1.212994990549,1.212994990549,1.212994990549,
1.212994990549,1.212994990549,1.212994990549,1.212994990549,1.212994990549,
1.212994990549,1.212994990549,1.212994990549),(0.9290016698171,0.9290016698171,
0.9290016698171,0.9290016698171,0.9290016698171,0.9290016698171,0.9290016698171,
0.9290016698171,0.9290016698171,0.9290016698171,0.9290016698171),(0.9290016698171,
0.9290016698171,0.9290016698171,0.9290016698171,0.9290016698171,0.9290016698171,
0.9290016698171,0.9290016698171,0.9290016698171,0.9290016698171,0.9290016698171),
(1.212994990549,1.212994990549,1.212994990549,1.212994990549,1.212994990549,
1.212994990549,1.212994990549,1.212994990549,1.212994990549,1.212994990549,
1.212994990549)))
REPRESENTATION_ITEM('')
SURFACE()
);
#866=(
BOUNDED_SURFACE()
B_SPLINE_SURFACE(3,3,((#50606,#50607,#50608,#50609,#50610,#50611,#50612,
#50613,#50614,#50615,#50616),(#50617,#50618,#50619,#50620,#50621,#50622,
#50623,#50624,#50625,#50626,#50627),(#50628,#50629,#50630,#50631,#50632,
#50633,#50634,#50635,#50636,#50637,#50638),(#50639,#50640,#50641,#50642,
#50643,#50644,#50645,#50646,#50647,#50648,#50649)),.UNSPECIFIED.,.F.,.F.,
 .F.)
B_SPLINE_SURFACE_WITH_KNOTS((4,4),(4,1,1,1,1,1,1,1,4),(0.,1.),(0.4912070765429,
0.5104451093027,0.5824328871872,0.6465099292207,0.7028608084679,0.7531387245365,
0.7991472729598,0.8414732732765,0.8528428231596),.UNSPECIFIED.)
GEOMETRIC_REPRESENTATION_ITEM()
RATIONAL_B_SPLINE_SURFACE(((1.212994990461,1.212994990461,1.212994990461,
1.212994990461,1.212994990461,1.212994990461,1.212994990461,1.212994990461,
1.212994990461,1.212994990461,1.212994990461),(0.9290016698463,0.9290016698463,
0.9290016698463,0.9290016698463,0.9290016698463,0.9290016698463,0.9290016698463,
0.9290016698463,0.9290016698463,0.9290016698463,0.9290016698463),(0.9290016698463,
0.9290016698463,0.9290016698463,0.9290016698463,0.9290016698463,0.9290016698463,
0.9290016698463,0.9290016698463,0.9290016698463,0.9290016698463,0.9290016698463),
(1.212994990461,1.212994990461,1.212994990461,1.212994990461,1.212994990461,
1.212994990461,1.212994990461,1.212994990461,1.212994990461,1.212994990461,
1.212994990461)))
REPRESENTATION_ITEM('')
SURFACE()
);
#867=(
BOUNDED_SURFACE()
B_SPLINE_SURFACE(3,3,((#50653,#50654,#50655,#50656,#50657,#50658,#50659,
#50660,#50661,#50662,#50663),(#50664,#50665,#50666,#50667,#50668,#50669,
#50670,#50671,#50672,#50673,#50674),(#50675,#50676,#50677,#50678,#50679,
#50680,#50681,#50682,#50683,#50684,#50685),(#50686,#50687,#50688,#50689,
#50690,#50691,#50692,#50693,#50694,#50695,#50696)),.UNSPECIFIED.,.F.,.F.,
 .F.)
B_SPLINE_SURFACE_WITH_KNOTS((4,4),(4,1,1,1,1,1,1,1,4),(0.,1.),(0.1471313081811,
0.1585267267235,0.2008527270402,0.2468612754635,0.2971391915321,0.3534900707793,
0.4175671128127,0.4895548906972,0.5087566656269),.UNSPECIFIED.)
GEOMETRIC_REPRESENTATION_ITEM()
RATIONAL_B_SPLINE_SURFACE(((1.212994990549,1.212994990549,1.212994990549,
1.212994990549,1.212994990549,1.212994990549,1.212994990549,1.212994990549,
1.212994990549,1.212994990549,1.212994990549),(0.9290016698171,0.9290016698171,
0.9290016698171,0.9290016698171,0.9290016698171,0.9290016698171,0.9290016698171,
0.9290016698171,0.9290016698171,0.9290016698171,0.9290016698171),(0.9290016698171,
0.9290016698171,0.9290016698171,0.9290016698171,0.9290016698171,0.9290016698171,
0.9290016698171,0.9290016698171,0.9290016698171,0.9290016698171,0.9290016698171),
(1.212994990549,1.212994990549,1.212994990549,1.212994990549,1.212994990549,
1.212994990549,1.212994990549,1.212994990549,1.212994990549,1.212994990549,
1.212994990549)))
REPRESENTATION_ITEM('')
SURFACE()
);
#868=(
BOUNDED_SURFACE()
B_SPLINE_SURFACE(3,3,((#50771,#50772,#50773,#50774,#50775,#50776,#50777,
#50778,#50779),(#50780,#50781,#50782,#50783,#50784,#50785,#50786,#50787,
#50788),(#50789,#50790,#50791,#50792,#50793,#50794,#50795,#50796,#50797),
(#50798,#50799,#50800,#50801,#50802,#50803,#50804,#50805,#50806)),
 .UNSPECIFIED.,.F.,.F.,.F.)
B_SPLINE_SURFACE_WITH_KNOTS((4,4),(4,1,1,1,1,1,4),(0.,1.),(0.1657200395971,
0.218898549315,0.2912491980128,0.3619657900993,0.4315535161345,0.500650977664,
0.5134507157828),.UNSPECIFIED.)
GEOMETRIC_REPRESENTATION_ITEM()
RATIONAL_B_SPLINE_SURFACE(((1.212996916314,1.212996916314,1.212996916314,
1.212996916314,1.212996916314,1.212996916314,1.212996916314,1.212996916314,
1.212996916314),(0.9290010278954,0.9290010278954,0.9290010278954,0.9290010278954,
0.9290010278954,0.9290010278954,0.9290010278954,0.9290010278954,0.9290010278954),
(0.9290010278954,0.9290010278954,0.9290010278954,0.9290010278954,0.9290010278954,
0.9290010278954,0.9290010278954,0.9290010278954,0.9290010278954),(1.212996916314,
1.212996916314,1.212996916314,1.212996916314,1.212996916314,1.212996916314,
1.212996916314,1.212996916314,1.212996916314)))
REPRESENTATION_ITEM('')
SURFACE()
);
#869=(
BOUNDED_SURFACE()
B_SPLINE_SURFACE(3,3,((#50824,#50825,#50826,#50827,#50828,#50829,#50830,
#50831,#50832,#50833,#50834),(#50835,#50836,#50837,#50838,#50839,#50840,
#50841,#50842,#50843,#50844,#50845),(#50846,#50847,#50848,#50849,#50850,
#50851,#50852,#50853,#50854,#50855,#50856),(#50857,#50858,#50859,#50860,
#50861,#50862,#50863,#50864,#50865,#50866,#50867)),.UNSPECIFIED.,.F.,.F.,
 .F.)
B_SPLINE_SURFACE_WITH_KNOTS((4,4),(4,1,1,1,1,1,1,1,4),(0.,1.),(0.1471313081811,
0.1585267267235,0.2008527270402,0.2468612754635,0.297139191532,0.3534900707792,
0.4175671128127,0.4895548906972,0.5087566656269),.UNSPECIFIED.)
GEOMETRIC_REPRESENTATION_ITEM()
RATIONAL_B_SPLINE_SURFACE(((1.212994990549,1.212994990549,1.212994990549,
1.212994990549,1.212994990549,1.212994990549,1.212994990549,1.212994990549,
1.212994990549,1.212994990549,1.212994990549),(0.9290016698171,0.9290016698171,
0.9290016698171,0.9290016698171,0.9290016698171,0.9290016698171,0.9290016698171,
0.9290016698171,0.9290016698171,0.9290016698171,0.9290016698171),(0.9290016698171,
0.9290016698171,0.9290016698171,0.9290016698171,0.9290016698171,0.9290016698171,
0.9290016698171,0.9290016698171,0.9290016698171,0.9290016698171,0.9290016698171),
(1.212994990549,1.212994990549,1.212994990549,1.212994990549,1.212994990549,
1.212994990549,1.212994990549,1.212994990549,1.212994990549,1.212994990549,
1.212994990549)))
REPRESENTATION_ITEM('')
SURFACE()
);
#874=TOROIDAL_SURFACE('',#34169,8.96,2.54);
#875=TOROIDAL_SURFACE('',#34194,49.79,2.54);
#876=TOROIDAL_SURFACE('',#34210,49.79,2.54);
#877=TOROIDAL_SURFACE('',#34231,8.96,2.54);
#878=TOROIDAL_SURFACE('',#34239,8.96,2.54);
#879=TOROIDAL_SURFACE('',#34256,49.79,2.54);
#880=TOROIDAL_SURFACE('',#34276,49.79,2.54);
#881=TOROIDAL_SURFACE('',#34281,49.79,2.54);
#882=TOROIDAL_SURFACE('',#34296,8.96,2.54);
#883=TOROIDAL_SURFACE('',#34310,49.79,2.54);
#884=TOROIDAL_SURFACE('',#34335,49.79,2.54);
#885=TOROIDAL_SURFACE('',#34337,49.79,2.54);
#886=TOROIDAL_SURFACE('',#34344,44.71,2.54);
#887=TOROIDAL_SURFACE('',#34349,38.29,2.54);
#912=SHAPE_REPRESENTATION_RELATIONSHIP('SRR','None',#61970,#937);
#937=ADVANCED_BREP_SHAPE_REPRESENTATION('',(#1001),#61783);
#962=STYLED_ITEM('',(#62156),#1001);
#1001=MANIFOLD_SOLID_BREP('Body1',#33792);
#1045=CYLINDRICAL_SURFACE('',#34167,11.5);
#1046=CYLINDRICAL_SURFACE('',#34173,2.54);
#1047=CYLINDRICAL_SURFACE('',#34190,5.75);
#1048=CYLINDRICAL_SURFACE('',#34191,5.75);
#1049=CYLINDRICAL_SURFACE('',#34192,5.75);
#1050=CYLINDRICAL_SURFACE('',#34193,5.75);
#1051=CYLINDRICAL_SURFACE('',#34199,47.25);
#1052=CYLINDRICAL_SURFACE('',#34221,2.54);
#1053=CYLINDRICAL_SURFACE('',#34224,2.54);
#1054=CYLINDRICAL_SURFACE('',#34229,2.54);
#1055=CYLINDRICAL_SURFACE('',#34234,11.5);
#1056=CYLINDRICAL_SURFACE('',#34236,2.54);
#1057=CYLINDRICAL_SURFACE('',#34242,11.5);
#1058=CYLINDRICAL_SURFACE('',#34245,2.54);
#1059=CYLINDRICAL_SURFACE('',#34251,2.54);
#1060=CYLINDRICAL_SURFACE('',#34255,2.54);
#1061=CYLINDRICAL_SURFACE('',#34259,2.54);
#1062=CYLINDRICAL_SURFACE('',#34264,2.54);
#1063=CYLINDRICAL_SURFACE('',#34266,2.54);
#1064=CYLINDRICAL_SURFACE('',#34271,2.54);
#1065=CYLINDRICAL_SURFACE('',#34275,2.54);
#1066=CYLINDRICAL_SURFACE('',#34280,2.54);
#1067=CYLINDRICAL_SURFACE('',#34285,2.54);
#1068=CYLINDRICAL_SURFACE('',#34287,2.54);
#1069=CYLINDRICAL_SURFACE('',#34291,2.54);
#1070=CYLINDRICAL_SURFACE('',#34294,11.5);
#1071=CYLINDRICAL_SURFACE('',#34299,2.54);
#1072=CYLINDRICAL_SURFACE('',#34302,2.54);
#1073=CYLINDRICAL_SURFACE('',#34307,2.54);
#1074=CYLINDRICAL_SURFACE('',#34313,2.54);
#1075=CYLINDRICAL_SURFACE('',#34318,2.54);
#1076=CYLINDRICAL_SURFACE('',#34319,2.54);
#1077=CYLINDRICAL_SURFACE('',#34325,2.54);
#1078=CYLINDRICAL_SURFACE('',#34327,2.54);
#1079=CYLINDRICAL_SURFACE('',#34330,2.54);
#1080=CYLINDRICAL_SURFACE('',#34338,2.54);
#1081=CYLINDRICAL_SURFACE('',#34341,2.54);
#1082=CYLINDRICAL_SURFACE('',#34353,35.75);
#1083=CYLINDRICAL_SURFACE('',#34357,27.315);
#1084=CYLINDRICAL_SURFACE('',#34361,23.435);
#1085=CYLINDRICAL_SURFACE('',#34365,15.);
#1086=CYLINDRICAL_SURFACE('',#34369,23.435);
#1087=CYLINDRICAL_SURFACE('',#34373,27.315);
#1088=CYLINDRICAL_SURFACE('',#34377,35.75);
#1089=CYLINDRICAL_SURFACE('',#34384,11.5);
#1090=CYLINDRICAL_SURFACE('',#34386,11.5);
#1091=CYLINDRICAL_SURFACE('',#34388,11.5);
#1092=CYLINDRICAL_SURFACE('',#34390,11.5);
#1880=FACE_BOUND('',#6134,.T.);
#1881=FACE_BOUND('',#6135,.T.);
#1882=FACE_BOUND('',#6136,.T.);
#1883=FACE_BOUND('',#6137,.T.);
#1884=FACE_BOUND('',#6138,.T.);
#1885=FACE_BOUND('',#6143,.T.);
#1886=FACE_BOUND('',#6145,.T.);
#1887=FACE_BOUND('',#6147,.T.);
#1888=FACE_BOUND('',#6149,.T.);
#1889=FACE_BOUND('',#6238,.T.);
#1890=FACE_BOUND('',#6242,.T.);
#1891=FACE_BOUND('',#6245,.T.);
#1892=FACE_BOUND('',#6248,.T.);
#1893=FACE_BOUND('',#6251,.T.);
#1894=FACE_BOUND('',#6254,.T.);
#1895=FACE_BOUND('',#6257,.T.);
#1896=FACE_BOUND('',#6260,.T.);
#2250=CIRCLE('',#34155,11.5);
#2251=CIRCLE('',#34156,11.5);
#2252=CIRCLE('',#34157,11.5);
#2253=CIRCLE('',#34158,11.5);
#2254=CIRCLE('',#34159,5.75);
#2255=CIRCLE('',#34160,5.75);
#2256=CIRCLE('',#34161,5.75);
#2257=CIRCLE('',#34162,5.75);
#2258=CIRCLE('',#34163,11.5);
#2259=CIRCLE('',#34164,11.5);
#2260=CIRCLE('',#34165,11.5);
#2261=CIRCLE('',#34166,11.5);
#2262=CIRCLE('',#34168,11.5);
#2263=CIRCLE('',#34170,2.54);
#2264=CIRCLE('',#34171,8.960000684551);
#2265=CIRCLE('',#34172,2.54);
#2266=CIRCLE('',#34174,2.54);
#2267=CIRCLE('',#34176,49.78996319131);
#2268=CIRCLE('',#34177,8.960000684551);
#2269=CIRCLE('',#34178,5.75);
#2270=CIRCLE('',#34180,49.78996141255);
#2271=CIRCLE('',#34181,8.960000684551);
#2272=CIRCLE('',#34182,5.75);
#2273=CIRCLE('',#34184,49.78996319131);
#2274=CIRCLE('',#34185,5.75);
#2275=CIRCLE('',#34187,49.78996141255);
#2276=CIRCLE('',#34188,8.960000684551);
#2277=CIRCLE('',#34189,5.75);
#2278=CIRCLE('',#34195,2.539999943211);
#2279=CIRCLE('',#34196,47.25);
#2280=CIRCLE('',#34197,2.54);
#2281=CIRCLE('',#34198,2.539975517689);
#2282=CIRCLE('',#34200,47.25);
#2283=CIRCLE('',#34201,47.25);
#2284=CIRCLE('',#34202,47.25);
#2285=CIRCLE('',#34203,47.25);
#2286=CIRCLE('',#34204,47.25);
#2287=CIRCLE('',#34205,47.25);
#2288=CIRCLE('',#34206,47.25);
#2289=CIRCLE('',#34207,47.25);
#2290=CIRCLE('',#34208,47.25);
#2291=CIRCLE('',#34209,47.25);
#2292=CIRCLE('',#34211,49.79);
#2293=CIRCLE('',#34212,2.54);
#2294=CIRCLE('',#34213,2.54);
#2295=CIRCLE('',#34216,49.79);
#2296=CIRCLE('',#34218,49.79);
#2297=CIRCLE('',#34220,49.79);
#2298=CIRCLE('',#34222,2.54);
#2299=CIRCLE('',#34225,2.54);
#2300=CIRCLE('',#34227,2.539999283673);
#2301=CIRCLE('',#34228,2.54);
#2302=CIRCLE('',#34230,2.54);
#2303=CIRCLE('',#34232,11.5);
#2304=CIRCLE('',#34233,2.54);
#2305=CIRCLE('',#34237,2.54);
#2306=CIRCLE('',#34238,2.54);
#2307=CIRCLE('',#34240,11.5);
#2308=CIRCLE('',#34241,2.54);
#2309=CIRCLE('',#34244,2.540003327809);
#2310=CIRCLE('',#34246,2.54);
#2311=CIRCLE('',#34248,2.54);
#2312=CIRCLE('',#34249,2.539975498399);
#2313=CIRCLE('',#34250,2.539999989149);
#2314=CIRCLE('',#34252,2.54);
#2315=CIRCLE('',#34254,2.54);
#2316=CIRCLE('',#34257,2.54);
#2317=CIRCLE('',#34258,2.539975299827);
#2318=CIRCLE('',#34260,2.54);
#2319=CIRCLE('',#34262,2.539999283673);
#2320=CIRCLE('',#34263,2.54);
#2321=CIRCLE('',#34265,2.540003327809);
#2322=CIRCLE('',#34267,2.54);
#2323=CIRCLE('',#34269,2.54);
#2324=CIRCLE('',#34270,2.539975344705);
#2325=CIRCLE('',#34272,2.54);
#2326=CIRCLE('',#34274,2.54);
#2327=CIRCLE('',#34277,2.54);
#2328=CIRCLE('',#34279,2.54);
#2329=CIRCLE('',#34282,2.54);
#2330=CIRCLE('',#34283,2.539975498399);
#2331=CIRCLE('',#34284,2.539999989149);
#2332=CIRCLE('',#34286,2.54);
#2333=CIRCLE('',#34288,2.54);
#2334=CIRCLE('',#34290,2.540003327809);
#2335=CIRCLE('',#34292,2.54);
#2336=CIRCLE('',#34295,11.5);
#2337=CIRCLE('',#34297,2.54);
#2338=CIRCLE('',#34298,2.54);
#2339=CIRCLE('',#34300,2.54);
#2340=CIRCLE('',#34303,2.54);
#2341=CIRCLE('',#34305,2.54);
#2342=CIRCLE('',#34306,2.539999283994);
#2343=CIRCLE('',#34308,2.539975344705);
#2344=CIRCLE('',#34309,2.539999943211);
#2345=CIRCLE('',#34311,2.54);
#2346=CIRCLE('',#34312,2.539975517689);
#2347=CIRCLE('',#34314,2.54);
#2348=CIRCLE('',#34316,2.539999283673);
#2349=CIRCLE('',#34317,2.54);
#2350=CIRCLE('',#34320,2.54);
#2351=CIRCLE('',#34323,2.54);
#2352=CIRCLE('',#34324,2.54);
#2353=CIRCLE('',#34326,2.540003327809);
#2354=CIRCLE('',#34328,2.54);
#2355=CIRCLE('',#34329,2.539999283673);
#2356=CIRCLE('',#34331,2.54);
#2357=CIRCLE('',#34333,2.53997529983);
#2358=CIRCLE('',#34334,2.54);
#2359=CIRCLE('',#34336,2.54);
#2360=CIRCLE('',#34339,2.54);
#2361=CIRCLE('',#34342,2.54);
#2362=CIRCLE('',#34345,44.70999983335);
#2363=CIRCLE('',#34346,2.54);
#2364=CIRCLE('',#34348,38.28999862038);
#2365=CIRCLE('',#34350,35.75);
#2366=CIRCLE('',#34351,35.75);
#2367=CIRCLE('',#34352,2.54);
#2368=CIRCLE('',#34354,35.75);
#2369=CIRCLE('',#34356,27.315);
#2370=CIRCLE('',#34358,27.315);
#2371=CIRCLE('',#34360,23.435);
#2372=CIRCLE('',#34362,23.435);
#2373=CIRCLE('',#34364,15.);
#2374=CIRCLE('',#34366,15.);
#2375=CIRCLE('',#34368,23.435);
#2376=CIRCLE('',#34370,23.435);
#2377=CIRCLE('',#34372,27.315);
#2378=CIRCLE('',#34374,27.315);
#2379=CIRCLE('',#34376,35.75);
#2380=CIRCLE('',#34378,35.75);
#2381=CIRCLE('',#34380,11.5);
#2382=CIRCLE('',#34381,11.5);
#2383=CIRCLE('',#34382,11.5);
#2384=CIRCLE('',#34383,11.5);
#4253=FACE_OUTER_BOUND('',#6133,.T.);
#4254=FACE_OUTER_BOUND('',#6139,.T.);
#4255=FACE_OUTER_BOUND('',#6140,.T.);
#4256=FACE_OUTER_BOUND('',#6141,.T.);
#4257=FACE_OUTER_BOUND('',#6142,.T.);
#4258=FACE_OUTER_BOUND('',#6144,.T.);
#4259=FACE_OUTER_BOUND('',#6146,.T.);
#4260=FACE_OUTER_BOUND('',#6148,.T.);
#4261=FACE_OUTER_BOUND('',#6150,.T.);
#4262=FACE_OUTER_BOUND('',#6151,.T.);
#4263=FACE_OUTER_BOUND('',#6152,.T.);
#4264=FACE_OUTER_BOUND('',#6153,.T.);
#4265=FACE_OUTER_BOUND('',#6154,.T.);
#4266=FACE_OUTER_BOUND('',#6155,.T.);
#4267=FACE_OUTER_BOUND('',#6156,.T.);
#4268=FACE_OUTER_BOUND('',#6157,.T.);
#4269=FACE_OUTER_BOUND('',#6158,.T.);
#4270=FACE_OUTER_BOUND('',#6159,.T.);
#4271=FACE_OUTER_BOUND('',#6160,.T.);
#4272=FACE_OUTER_BOUND('',#6161,.T.);
#4273=FACE_OUTER_BOUND('',#6162,.T.);
#4274=FACE_OUTER_BOUND('',#6163,.T.);
#4275=FACE_OUTER_BOUND('',#6164,.T.);
#4276=FACE_OUTER_BOUND('',#6165,.T.);
#4277=FACE_OUTER_BOUND('',#6166,.T.);
#4278=FACE_OUTER_BOUND('',#6167,.T.);
#4279=FACE_OUTER_BOUND('',#6168,.T.);
#4280=FACE_OUTER_BOUND('',#6169,.T.);
#4281=FACE_OUTER_BOUND('',#6170,.T.);
#4282=FACE_OUTER_BOUND('',#6171,.T.);
#4283=FACE_OUTER_BOUND('',#6172,.T.);
#4284=FACE_OUTER_BOUND('',#6173,.T.);
#4285=FACE_OUTER_BOUND('',#6174,.T.);
#4286=FACE_OUTER_BOUND('',#6175,.T.);
#4287=FACE_OUTER_BOUND('',#6176,.T.);
#4288=FACE_OUTER_BOUND('',#6177,.T.);
#4289=FACE_OUTER_BOUND('',#6178,.T.);
#4290=FACE_OUTER_BOUND('',#6179,.T.);
#4291=FACE_OUTER_BOUND('',#6180,.T.);
#4292=FACE_OUTER_BOUND('',#6181,.T.);
#4293=FACE_OUTER_BOUND('',#6182,.T.);
#4294=FACE_OUTER_BOUND('',#6183,.T.);
#4295=FACE_OUTER_BOUND('',#6184,.T.);
#4296=FACE_OUTER_BOUND('',#6185,.T.);
#4297=FACE_OUTER_BOUND('',#6186,.T.);
#4298=FACE_OUTER_BOUND('',#6187,.T.);
#4299=FACE_OUTER_BOUND('',#6188,.T.);
#4300=FACE_OUTER_BOUND('',#6189,.T.);
#4301=FACE_OUTER_BOUND('',#6190,.T.);
#4302=FACE_OUTER_BOUND('',#6191,.T.);
#4303=FACE_OUTER_BOUND('',#6192,.T.);
#4304=FACE_OUTER_BOUND('',#6193,.T.);
#4305=FACE_OUTER_BOUND('',#6194,.T.);
#4306=FACE_OUTER_BOUND('',#6195,.T.);
#4307=FACE_OUTER_BOUND('',#6196,.T.);
#4308=FACE_OUTER_BOUND('',#6197,.T.);
#4309=FACE_OUTER_BOUND('',#6198,.T.);
#4310=FACE_OUTER_BOUND('',#6199,.T.);
#4311=FACE_OUTER_BOUND('',#6200,.T.);
#4312=FACE_OUTER_BOUND('',#6201,.T.);
#4313=FACE_OUTER_BOUND('',#6202,.T.);
#4314=FACE_OUTER_BOUND('',#6203,.T.);
#4315=FACE_OUTER_BOUND('',#6204,.T.);
#4316=FACE_OUTER_BOUND('',#6205,.T.);
#4317=FACE_OUTER_BOUND('',#6206,.T.);
#4318=FACE_OUTER_BOUND('',#6207,.T.);
#4319=FACE_OUTER_BOUND('',#6208,.T.);
#4320=FACE_OUTER_BOUND('',#6209,.T.);
#4321=FACE_OUTER_BOUND('',#6210,.T.);
#4322=FACE_OUTER_BOUND('',#6211,.T.);
#4323=FACE_OUTER_BOUND('',#6212,.T.);
#4324=FACE_OUTER_BOUND('',#6213,.T.);
#4325=FACE_OUTER_BOUND('',#6214,.T.);
#4326=FACE_OUTER_BOUND('',#6215,.T.);
#4327=FACE_OUTER_BOUND('',#6216,.T.);
#4328=FACE_OUTER_BOUND('',#6217,.T.);
#4329=FACE_OUTER_BOUND('',#6218,.T.);
#4330=FACE_OUTER_BOUND('',#6219,.T.);
#4331=FACE_OUTER_BOUND('',#6220,.T.);
#4332=FACE_OUTER_BOUND('',#6221,.T.);
#4333=FACE_OUTER_BOUND('',#6222,.T.);
#4334=FACE_OUTER_BOUND('',#6223,.T.);
#4335=FACE_OUTER_BOUND('',#6224,.T.);
#4336=FACE_OUTER_BOUND('',#6225,.T.);
#4337=FACE_OUTER_BOUND('',#6226,.T.);
#4338=FACE_OUTER_BOUND('',#6227,.T.);
#4339=FACE_OUTER_BOUND('',#6228,.T.);
#4340=FACE_OUTER_BOUND('',#6229,.T.);
#4341=FACE_OUTER_BOUND('',#6230,.T.);
#4342=FACE_OUTER_BOUND('',#6231,.T.);
#4343=FACE_OUTER_BOUND('',#6232,.T.);
#4344=FACE_OUTER_BOUND('',#6233,.T.);
#4345=FACE_OUTER_BOUND('',#6234,.T.);
#4346=FACE_OUTER_BOUND('',#6235,.T.);
#4347=FACE_OUTER_BOUND('',#6236,.T.);
#4348=FACE_OUTER_BOUND('',#6237,.T.);
#4349=FACE_OUTER_BOUND('',#6239,.T.);
#4350=FACE_OUTER_BOUND('',#6240,.T.);
#4351=FACE_OUTER_BOUND('',#6241,.T.);
#4352=FACE_OUTER_BOUND('',#6243,.T.);
#4353=FACE_OUTER_BOUND('',#6244,.T.);
#4354=FACE_OUTER_BOUND('',#6246,.T.);
#4355=FACE_OUTER_BOUND('',#6247,.T.);
#4356=FACE_OUTER_BOUND('',#6249,.T.);
#4357=FACE_OUTER_BOUND('',#6250,.T.);
#4358=FACE_OUTER_BOUND('',#6252,.T.);
#4359=FACE_OUTER_BOUND('',#6253,.T.);
#4360=FACE_OUTER_BOUND('',#6255,.T.);
#4361=FACE_OUTER_BOUND('',#6256,.T.);
#4362=FACE_OUTER_BOUND('',#6258,.T.);
#4363=FACE_OUTER_BOUND('',#6259,.T.);
#4364=FACE_OUTER_BOUND('',#6261,.T.);
#4365=FACE_OUTER_BOUND('',#6262,.T.);
#4366=FACE_OUTER_BOUND('',#6263,.T.);
#4367=FACE_OUTER_BOUND('',#6264,.T.);
#4368=FACE_OUTER_BOUND('',#6265,.T.);
#4369=FACE_OUTER_BOUND('',#6266,.T.);
#4370=FACE_OUTER_BOUND('',#6267,.T.);
#4371=FACE_OUTER_BOUND('',#6268,.T.);
#6133=EDGE_LOOP('',(#21572,#21573,#21574,#21575,#21576,#21577,#21578,#21579));
#6134=EDGE_LOOP('',(#21580));
#6135=EDGE_LOOP('',(#21581));
#6136=EDGE_LOOP('',(#21582));
#6137=EDGE_LOOP('',(#21583));
#6138=EDGE_LOOP('',(#21584,#21585,#21586,#21587,#21588,#21589,#21590,#21591));
#6139=EDGE_LOOP('',(#21592,#21593,#21594,#21595));
#6140=EDGE_LOOP('',(#21596,#21597,#21598,#21599));
#6141=EDGE_LOOP('',(#21600,#21601,#21602,#21603));
#6142=EDGE_LOOP('',(#21604,#21605,#21606,#21607,#21608,#21609));
#6143=EDGE_LOOP('',(#21610));
#6144=EDGE_LOOP('',(#21611,#21612,#21613,#21614,#21615,#21616));
#6145=EDGE_LOOP('',(#21617));
#6146=EDGE_LOOP('',(#21618,#21619,#21620,#21621,#21622,#21623));
#6147=EDGE_LOOP('',(#21624));
#6148=EDGE_LOOP('',(#21625,#21626,#21627,#21628,#21629,#21630));
#6149=EDGE_LOOP('',(#21631));
#6150=EDGE_LOOP('',(#21632,#21633,#21634,#21635));
#6151=EDGE_LOOP('',(#21636,#21637,#21638,#21639));
#6152=EDGE_LOOP('',(#21640,#21641,#21642,#21643));
#6153=EDGE_LOOP('',(#21644,#21645,#21646,#21647));
#6154=EDGE_LOOP('',(#21648,#21649,#21650,#21651));
#6155=EDGE_LOOP('',(#21652,#21653,#21654,#21655));
#6156=EDGE_LOOP('',(#21656,#21657,#21658,#21659,#21660,#21661,#21662,#21663,
#21664,#21665,#21666,#21667,#21668,#21669,#21670,#21671,#21672,#21673,#21674,
#21675,#21676));
#6157=EDGE_LOOP('',(#21677,#21678,#21679,#21680,#21681));
#6158=EDGE_LOOP('',(#21682,#21683,#21684,#21685));
#6159=EDGE_LOOP('',(#21686,#21687,#21688,#21689));
#6160=EDGE_LOOP('',(#21690,#21691,#21692,#21693));
#6161=EDGE_LOOP('',(#21694,#21695,#21696,#21697));
#6162=EDGE_LOOP('',(#21698,#21699,#21700,#21701));
#6163=EDGE_LOOP('',(#21702,#21703,#21704));
#6164=EDGE_LOOP('',(#21705,#21706,#21707,#21708));
#6165=EDGE_LOOP('',(#21709,#21710,#21711));
#6166=EDGE_LOOP('',(#21712,#21713,#21714,#21715));
#6167=EDGE_LOOP('',(#21716,#21717,#21718,#21719));
#6168=EDGE_LOOP('',(#21720,#21721,#21722,#21723));
#6169=EDGE_LOOP('',(#21724,#21725,#21726,#21727,#21728,#21729,#21730,#21731));
#6170=EDGE_LOOP('',(#21732,#21733,#21734,#21735));
#6171=EDGE_LOOP('',(#21736,#21737,#21738,#21739));
#6172=EDGE_LOOP('',(#21740,#21741,#21742,#21743));
#6173=EDGE_LOOP('',(#21744,#21745,#21746,#21747,#21748,#21749,#21750,#21751));
#6174=EDGE_LOOP('',(#21752,#21753,#21754,#21755));
#6175=EDGE_LOOP('',(#21756,#21757,#21758,#21759));
#6176=EDGE_LOOP('',(#21760,#21761,#21762));
#6177=EDGE_LOOP('',(#21763,#21764,#21765,#21766));
#6178=EDGE_LOOP('',(#21767,#21768,#21769,#21770));
#6179=EDGE_LOOP('',(#21771,#21772,#21773));
#6180=EDGE_LOOP('',(#21774,#21775,#21776,#21777));
#6181=EDGE_LOOP('',(#21778,#21779,#21780,#21781));
#6182=EDGE_LOOP('',(#21782,#21783,#21784,#21785));
#6183=EDGE_LOOP('',(#21786,#21787,#21788,#21789));
#6184=EDGE_LOOP('',(#21790,#21791,#21792));
#6185=EDGE_LOOP('',(#21793,#21794,#21795,#21796));
#6186=EDGE_LOOP('',(#21797,#21798,#21799,#21800));
#6187=EDGE_LOOP('',(#21801,#21802,#21803,#21804));
#6188=EDGE_LOOP('',(#21805,#21806,#21807,#21808));
#6189=EDGE_LOOP('',(#21809,#21810,#21811));
#6190=EDGE_LOOP('',(#21812,#21813,#21814,#21815));
#6191=EDGE_LOOP('',(#21816,#21817,#21818,#21819));
#6192=EDGE_LOOP('',(#21820,#21821,#21822));
#6193=EDGE_LOOP('',(#21823,#21824,#21825,#21826));
#6194=EDGE_LOOP('',(#21827,#21828,#21829,#21830));
#6195=EDGE_LOOP('',(#21831,#21832,#21833));
#6196=EDGE_LOOP('',(#21834,#21835,#21836,#21837));
#6197=EDGE_LOOP('',(#21838,#21839,#21840,#21841));
#6198=EDGE_LOOP('',(#21842,#21843,#21844,#21845));
#6199=EDGE_LOOP('',(#21846,#21847,#21848,#21849));
#6200=EDGE_LOOP('',(#21850,#21851,#21852,#21853));
#6201=EDGE_LOOP('',(#21854,#21855,#21856));
#6202=EDGE_LOOP('',(#21857,#21858,#21859,#21860));
#6203=EDGE_LOOP('',(#21861,#21862,#21863,#21864));
#6204=EDGE_LOOP('',(#21865,#21866,#21867,#21868,#21869,#21870,#21871,#21872));
#6205=EDGE_LOOP('',(#21873,#21874,#21875,#21876));
#6206=EDGE_LOOP('',(#21877,#21878,#21879,#21880));
#6207=EDGE_LOOP('',(#21881,#21882,#21883,#21884));
#6208=EDGE_LOOP('',(#21885,#21886,#21887,#21888,#21889,#21890,#21891,#21892));
#6209=EDGE_LOOP('',(#21893,#21894,#21895,#21896));
#6210=EDGE_LOOP('',(#21897,#21898,#21899));
#6211=EDGE_LOOP('',(#21900,#21901,#21902,#21903));
#6212=EDGE_LOOP('',(#21904,#21905,#21906,#21907));
#6213=EDGE_LOOP('',(#21908,#21909,#21910,#21911));
#6214=EDGE_LOOP('',(#21912,#21913,#21914,#21915));
#6215=EDGE_LOOP('',(#21916,#21917,#21918,#21919));
#6216=EDGE_LOOP('',(#21920,#21921,#21922));
#6217=EDGE_LOOP('',(#21923,#21924,#21925,#21926));
#6218=EDGE_LOOP('',(#21927,#21928,#21929,#21930));
#6219=EDGE_LOOP('',(#21931,#21932,#21933,#21934));
#6220=EDGE_LOOP('',(#21935,#21936,#21937));
#6221=EDGE_LOOP('',(#21938,#21939,#21940));
#6222=EDGE_LOOP('',(#21941,#21942,#21943,#21944));
#6223=EDGE_LOOP('',(#21945,#21946,#21947,#21948));
#6224=EDGE_LOOP('',(#21949,#21950,#21951,#21952));
#6225=EDGE_LOOP('',(#21953,#21954,#21955,#21956));
#6226=EDGE_LOOP('',(#21957,#21958,#21959,#21960));
#6227=EDGE_LOOP('',(#21961,#21962,#21963));
#6228=EDGE_LOOP('',(#21964,#21965,#21966,#21967));
#6229=EDGE_LOOP('',(#21968,#21969,#21970,#21971));
#6230=EDGE_LOOP('',(#21972,#21973,#21974,#21975));
#6231=EDGE_LOOP('',(#21976,#21977,#21978,#21979));
#6232=EDGE_LOOP('',(#21980,#21981,#21982));
#6233=EDGE_LOOP('',(#21983,#21984,#21985,#21986));
#6234=EDGE_LOOP('',(#21987,#21988,#21989));
#6235=EDGE_LOOP('',(#21990,#21991,#21992,#21993));
#6236=EDGE_LOOP('',(#21994,#21995,#21996,#21997,#21998));
#6237=EDGE_LOOP('',(#21999));
#6238=EDGE_LOOP('',(#22000));
#6239=EDGE_LOOP('',(#22001,#22002,#22003,#22004,#22005));
#6240=EDGE_LOOP('',(#22006,#22007,#22008,#22009,#22010));
#6241=EDGE_LOOP('',(#22011));
#6242=EDGE_LOOP('',(#22012));
#6243=EDGE_LOOP('',(#22013,#22014,#22015,#22016));
#6244=EDGE_LOOP('',(#22017));
#6245=EDGE_LOOP('',(#22018));
#6246=EDGE_LOOP('',(#22019,#22020,#22021,#22022));
#6247=EDGE_LOOP('',(#22023));
#6248=EDGE_LOOP('',(#22024));
#6249=EDGE_LOOP('',(#22025,#22026,#22027,#22028));
#6250=EDGE_LOOP('',(#22029));
#6251=EDGE_LOOP('',(#22030));
#6252=EDGE_LOOP('',(#22031,#22032,#22033,#22034));
#6253=EDGE_LOOP('',(#22035));
#6254=EDGE_LOOP('',(#22036));
#6255=EDGE_LOOP('',(#22037,#22038,#22039,#22040));
#6256=EDGE_LOOP('',(#22041));
#6257=EDGE_LOOP('',(#22042));
#6258=EDGE_LOOP('',(#22043,#22044,#22045,#22046));
#6259=EDGE_LOOP('',(#22047,#22048,#22049,#22050,#22051,#22052,#22053,#22054));
#6260=EDGE_LOOP('',(#22055));
#6261=EDGE_LOOP('',(#22056,#22057,#22058,#22059));
#6262=EDGE_LOOP('',(#22060,#22061,#22062,#22063));
#6263=EDGE_LOOP('',(#22064,#22065,#22066,#22067));
#6264=EDGE_LOOP('',(#22068,#22069,#22070,#22071));
#6265=EDGE_LOOP('',(#22072,#22073,#22074,#22075));
#6266=EDGE_LOOP('',(#22076,#22077,#22078,#22079));
#6267=EDGE_LOOP('',(#22080,#22081,#22082,#22083));
#6268=EDGE_LOOP('',(#22084,#22085,#22086,#22087));
#8389=LINE('',#48961,#10936);
#8390=LINE('',#48965,#10937);
#8391=LINE('',#48969,#10938);
#8392=LINE('',#48972,#10939);
#8393=LINE('',#48985,#10940);
#8394=LINE('',#48989,#10941);
#8395=LINE('',#48993,#10942);
#8396=LINE('',#48996,#10943);
#8397=LINE('',#49001,#10944);
#8398=LINE('',#49002,#10945);
#8399=LINE('',#49011,#10946);
#8400=LINE('',#49014,#10947);
#8401=LINE('',#49020,#10948);
#8402=LINE('',#49022,#10949);
#8403=LINE('',#49026,#10950);
#8404=LINE('',#49027,#10951);
#8405=LINE('',#49035,#10952);
#8406=LINE('',#49037,#10953);
#8407=LINE('',#49041,#10954);
#8408=LINE('',#49042,#10955);
#8409=LINE('',#49049,#10956);
#8410=LINE('',#49051,#10957);
#8411=LINE('',#49052,#10958);
#8412=LINE('',#49060,#10959);
#8413=LINE('',#49062,#10960);
#8414=LINE('',#49066,#10961);
#8415=LINE('',#49067,#10962);
#8416=LINE('',#49071,#10963);
#8417=LINE('',#49073,#10964);
#8418=LINE('',#49075,#10965);
#8419=LINE('',#49077,#10966);
#8420=LINE('',#49159,#10967);
#8421=LINE('',#49253,#10968);
#8422=LINE('',#49255,#10969);
#8423=LINE('',#49256,#10970);
#8424=LINE('',#49262,#10971);
#8425=LINE('',#49264,#10972);
#8426=LINE('',#49265,#10973);
#8427=LINE('',#49271,#10974);
#8428=LINE('',#49273,#10975);
#8429=LINE('',#49274,#10976);
#8430=LINE('',#49280,#10977);
#8431=LINE('',#49282,#10978);
#8432=LINE('',#49283,#10979);
#8433=LINE('',#49342,#10980);
#8434=LINE('',#49352,#10981);
#8435=LINE('',#49359,#10982);
#8436=LINE('',#49360,#10983);
#8437=LINE('',#49364,#10984);
#8438=LINE('',#49377,#10985);
#8439=LINE('',#49389,#10986);
#8440=LINE('',#49390,#10987);
#8441=LINE('',#49399,#10988);
#8442=LINE('',#49413,#10989);
#8443=LINE('',#49425,#10990);
#8444=LINE('',#49582,#10991);
#8445=LINE('',#49701,#10992);
#8446=LINE('',#49971,#10993);
#8447=LINE('',#50096,#10994);
#8448=LINE('',#50257,#10995);
#8449=LINE('',#50271,#10996);
#8450=LINE('',#50272,#10997);
#8451=LINE('',#50276,#10998);
#8452=LINE('',#50283,#10999);
#8453=LINE('',#50297,#11000);
#8454=LINE('',#50309,#11001);
#8455=LINE('',#50327,#11002);
#8456=LINE('',#50430,#11003);
#8457=LINE('',#50766,#11004);
#8458=LINE('',#50884,#11005);
#8459=LINE('',#50891,#11006);
#8460=LINE('',#50898,#11007);
#8461=LINE('',#50905,#11008);
#8462=LINE('',#50912,#11009);
#8463=LINE('',#50919,#11010);
#8464=LINE('',#50926,#11011);
#8465=LINE('',#50932,#11012);
#8466=LINE('',#50936,#11013);
#8467=LINE('',#50940,#11014);
#8468=LINE('',#50943,#11015);
#8469=LINE('',#50945,#11016);
#8470=LINE('',#50946,#11017);
#8471=LINE('',#50948,#11018);
#8472=LINE('',#50950,#11019);
#8473=LINE('',#50952,#11020);
#8474=LINE('',#50954,#11021);
#8475=LINE('',#50956,#11022);
#8476=LINE('',#50958,#11023);
#10936=VECTOR('',#38297,85.);
#10937=VECTOR('',#38300,85.);
#10938=VECTOR('',#38303,85.);
#10939=VECTOR('',#38306,85.);
#10940=VECTOR('',#38317,60.);
#10941=VECTOR('',#38320,60.);
#10942=VECTOR('',#38323,60.);
#10943=VECTOR('',#38326,60.);
#10944=VECTOR('',#38331,13.46);
#10945=VECTOR('',#38332,13.46);
#10946=VECTOR('',#38343,6.406394945352);
#10947=VECTOR('',#38346,6.40650331130805);
#10948=VECTOR('',#38351,13.1015672783503);
#10949=VECTOR('',#38352,6.406394945352);
#10950=VECTOR('',#38355,6.406394945352);
#10951=VECTOR('',#38356,13.1015672783303);
#10952=VECTOR('',#38363,13.1015672783301);
#10953=VECTOR('',#38364,6.406394945352);
#10954=VECTOR('',#38367,6.406394945352);
#10955=VECTOR('',#38368,13.1015672783004);
#10956=VECTOR('',#38375,13.1015672783503);
#10957=VECTOR('',#38376,6.406394945352);
#10958=VECTOR('',#38377,13.1015672783303);
#10959=VECTOR('',#38384,13.1015672783301);
#10960=VECTOR('',#38385,6.406394945352);
#10961=VECTOR('',#38388,6.406394945352);
#10962=VECTOR('',#38389,13.1015672783004);
#10963=VECTOR('',#38394,5.75);
#10964=VECTOR('',#38397,5.75);
#10965=VECTOR('',#38400,5.75);
#10966=VECTOR('',#38403,5.75);
#10967=VECTOR('',#38418,47.25);
#10968=VECTOR('',#38447,10.1277288760101);
#10969=VECTOR('',#38448,60.8968295013);
#10970=VECTOR('',#38449,10.1277306467203);
#10971=VECTOR('',#38454,10.1275050058501);
#10972=VECTOR('',#38455,60.8968295013);
#10973=VECTOR('',#38456,10.1275545073903);
#10974=VECTOR('',#38461,10.1277288760101);
#10975=VECTOR('',#38462,60.8968295013);
#10976=VECTOR('',#38463,10.1277306467203);
#10977=VECTOR('',#38468,10.1275522165901);
#10978=VECTOR('',#38469,60.8968295013);
#10979=VECTOR('',#38470,10.1274976633303);
#10980=VECTOR('',#38475,13.6647791615402);
#10981=VECTOR('',#38490,6.40650331130805);
#10982=VECTOR('',#38501,13.46);
#10983=VECTOR('',#38502,13.46);
#10984=VECTOR('',#38505,6.40650331130805);
#10985=VECTOR('',#38506,60.89682950219);
#10986=VECTOR('',#38507,6.40650330990706);
#10987=VECTOR('',#38508,13.46);
#10988=VECTOR('',#38523,13.46);
#10989=VECTOR('',#38526,6.40650330990706);
#10990=VECTOR('',#38527,60.89682950219);
#10991=VECTOR('',#38534,13.6647800109101);
#10992=VECTOR('',#38561,13.6647772519894);
#10993=VECTOR('',#38578,13.6647772688202);
#10994=VECTOR('',#38617,13.6647800109101);
#10995=VECTOR('',#38628,60.89682950219);
#10996=VECTOR('',#38633,6.40650330990706);
#10997=VECTOR('',#38634,13.46);
#10998=VECTOR('',#38639,13.46);
#10999=VECTOR('',#38650,6.40650331130805);
#11000=VECTOR('',#38653,60.89682950219);
#11001=VECTOR('',#38654,6.40650330906005);
#11002=VECTOR('',#38667,13.6647772688694);
#11003=VECTOR('',#38680,13.6647791615402);
#11004=VECTOR('',#38717,13.6647772519099);
#11005=VECTOR('',#38764,35.75);
#11006=VECTOR('',#38773,27.315);
#11007=VECTOR('',#38782,23.435);
#11008=VECTOR('',#38791,15.);
#11009=VECTOR('',#38800,23.435);
#11010=VECTOR('',#38809,27.315);
#11011=VECTOR('',#38818,35.75);
#11012=VECTOR('',#38823,60.);
#11013=VECTOR('',#38826,60.);
#11014=VECTOR('',#38829,60.);
#11015=VECTOR('',#38832,60.);
#11016=VECTOR('',#38835,3.81);
#11017=VECTOR('',#38836,3.81);
#11018=VECTOR('',#38839,3.81);
#11019=VECTOR('',#38842,3.81);
#11020=VECTOR('',#38845,3.81);
#11021=VECTOR('',#38848,3.81);
#11022=VECTOR('',#38851,3.81);
#11023=VECTOR('',#38854,3.81);
#13478=VERTEX_POINT('',#48957);
#13479=VERTEX_POINT('',#48958);
#13480=VERTEX_POINT('',#48960);
#13481=VERTEX_POINT('',#48962);
#13482=VERTEX_POINT('',#48964);
#13483=VERTEX_POINT('',#48966);
#13484=VERTEX_POINT('',#48968);
#13485=VERTEX_POINT('',#48970);
#13486=VERTEX_POINT('',#48973);
#13487=VERTEX_POINT('',#48975);
#13488=VERTEX_POINT('',#48977);
#13489=VERTEX_POINT('',#48979);
#13490=VERTEX_POINT('',#48981);
#13491=VERTEX_POINT('',#48982);
#13492=VERTEX_POINT('',#48984);
#13493=VERTEX_POINT('',#48986);
#13494=VERTEX_POINT('',#48988);
#13495=VERTEX_POINT('',#48990);
#13496=VERTEX_POINT('',#48992);
#13497=VERTEX_POINT('',#48994);
#13498=VERTEX_POINT('',#48998);
#13499=VERTEX_POINT('',#48999);
#13500=VERTEX_POINT('',#49004);
#13501=VERTEX_POINT('',#49006);
#13502=VERTEX_POINT('',#49010);
#13503=VERTEX_POINT('',#49012);
#13504=VERTEX_POINT('',#49016);
#13505=VERTEX_POINT('',#49017);
#13506=VERTEX_POINT('',#49019);
#13507=VERTEX_POINT('',#49021);
#13508=VERTEX_POINT('',#49023);
#13509=VERTEX_POINT('',#49025);
#13510=VERTEX_POINT('',#49028);
#13511=VERTEX_POINT('',#49031);
#13512=VERTEX_POINT('',#49032);
#13513=VERTEX_POINT('',#49034);
#13514=VERTEX_POINT('',#49036);
#13515=VERTEX_POINT('',#49038);
#13516=VERTEX_POINT('',#49040);
#13517=VERTEX_POINT('',#49043);
#13518=VERTEX_POINT('',#49046);
#13519=VERTEX_POINT('',#49047);
#13520=VERTEX_POINT('',#49050);
#13521=VERTEX_POINT('',#49053);
#13522=VERTEX_POINT('',#49056);
#13523=VERTEX_POINT('',#49057);
#13524=VERTEX_POINT('',#49059);
#13525=VERTEX_POINT('',#49061);
#13526=VERTEX_POINT('',#49063);
#13527=VERTEX_POINT('',#49065);
#13528=VERTEX_POINT('',#49068);
#13529=VERTEX_POINT('',#49079);
#13530=VERTEX_POINT('',#49081);
#13531=VERTEX_POINT('',#49120);
#13532=VERTEX_POINT('',#49130);
#13533=VERTEX_POINT('',#49155);
#13534=VERTEX_POINT('',#49156);
#13535=VERTEX_POINT('',#49158);
#13536=VERTEX_POINT('',#49161);
#13537=VERTEX_POINT('',#49171);
#13538=VERTEX_POINT('',#49173);
#13539=VERTEX_POINT('',#49183);
#13540=VERTEX_POINT('',#49185);
#13541=VERTEX_POINT('',#49195);
#13542=VERTEX_POINT('',#49197);
#13543=VERTEX_POINT('',#49207);
#13544=VERTEX_POINT('',#49209);
#13545=VERTEX_POINT('',#49219);
#13546=VERTEX_POINT('',#49221);
#13547=VERTEX_POINT('',#49231);
#13548=VERTEX_POINT('',#49233);
#13549=VERTEX_POINT('',#49246);
#13550=VERTEX_POINT('',#49247);
#13551=VERTEX_POINT('',#49252);
#13552=VERTEX_POINT('',#49254);
#13553=VERTEX_POINT('',#49258);
#13554=VERTEX_POINT('',#49259);
#13555=VERTEX_POINT('',#49261);
#13556=VERTEX_POINT('',#49263);
#13557=VERTEX_POINT('',#49267);
#13558=VERTEX_POINT('',#49268);
#13559=VERTEX_POINT('',#49270);
#13560=VERTEX_POINT('',#49272);
#13561=VERTEX_POINT('',#49276);
#13562=VERTEX_POINT('',#49277);
#13563=VERTEX_POINT('',#49279);
#13564=VERTEX_POINT('',#49281);
#13565=VERTEX_POINT('',#49286);
#13566=VERTEX_POINT('',#49347);
#13567=VERTEX_POINT('',#49351);
#13568=VERTEX_POINT('',#49355);
#13569=VERTEX_POINT('',#49362);
#13570=VERTEX_POINT('',#49363);
#13571=VERTEX_POINT('',#49365);
#13572=VERTEX_POINT('',#49376);
#13573=VERTEX_POINT('',#49378);
#13574=VERTEX_POINT('',#49395);
#13575=VERTEX_POINT('',#49401);
#13576=VERTEX_POINT('',#49402);
#13577=VERTEX_POINT('',#49414);
#13578=VERTEX_POINT('',#49470);
#13579=VERTEX_POINT('',#49580);
#13580=VERTEX_POINT('',#49688);
#13581=VERTEX_POINT('',#49700);
#13582=VERTEX_POINT('',#49860);
#13583=VERTEX_POINT('',#49969);
#13584=VERTEX_POINT('',#50068);
#13585=VERTEX_POINT('',#50094);
#13586=VERTEX_POINT('',#50199);
#13587=VERTEX_POINT('',#50243);
#13588=VERTEX_POINT('',#50256);
#13589=VERTEX_POINT('',#50270);
#13590=VERTEX_POINT('',#50274);
#13591=VERTEX_POINT('',#50281);
#13592=VERTEX_POINT('',#50285);
#13593=VERTEX_POINT('',#50296);
#13594=VERTEX_POINT('',#50298);
#13595=VERTEX_POINT('',#50313);
#13596=VERTEX_POINT('',#50317);
#13597=VERTEX_POINT('',#50404);
#13598=VERTEX_POINT('',#50429);
#13599=VERTEX_POINT('',#50697);
#13600=VERTEX_POINT('',#50764);
#13601=VERTEX_POINT('',#50869);
#13602=VERTEX_POINT('',#50873);
#13603=VERTEX_POINT('',#50876);
#13604=VERTEX_POINT('',#50877);
#13605=VERTEX_POINT('',#50882);
#13606=VERTEX_POINT('',#50886);
#13607=VERTEX_POINT('',#50889);
#13608=VERTEX_POINT('',#50893);
#13609=VERTEX_POINT('',#50896);
#13610=VERTEX_POINT('',#50900);
#13611=VERTEX_POINT('',#50903);
#13612=VERTEX_POINT('',#50907);
#13613=VERTEX_POINT('',#50910);
#13614=VERTEX_POINT('',#50914);
#13615=VERTEX_POINT('',#50917);
#13616=VERTEX_POINT('',#50921);
#13617=VERTEX_POINT('',#50924);
#13618=VERTEX_POINT('',#50928);
#13619=VERTEX_POINT('',#50929);
#13620=VERTEX_POINT('',#50931);
#13621=VERTEX_POINT('',#50933);
#13622=VERTEX_POINT('',#50935);
#13623=VERTEX_POINT('',#50937);
#13624=VERTEX_POINT('',#50939);
#13625=VERTEX_POINT('',#50941);
#16688=EDGE_CURVE('',#13478,#13479,#2250,.T.);
#16689=EDGE_CURVE('',#13479,#13480,#8389,.T.);
#16690=EDGE_CURVE('',#13480,#13481,#2251,.T.);
#16691=EDGE_CURVE('',#13481,#13482,#8390,.T.);
#16692=EDGE_CURVE('',#13482,#13483,#2252,.T.);
#16693=EDGE_CURVE('',#13483,#13484,#8391,.T.);
#16694=EDGE_CURVE('',#13484,#13485,#2253,.T.);
#16695=EDGE_CURVE('',#13485,#13478,#8392,.T.);
#16696=EDGE_CURVE('',#13486,#13486,#2254,.T.);
#16697=EDGE_CURVE('',#13487,#13487,#2255,.T.);
#16698=EDGE_CURVE('',#13488,#13488,#2256,.T.);
#16699=EDGE_CURVE('',#13489,#13489,#2257,.T.);
#16700=EDGE_CURVE('',#13490,#13491,#2258,.T.);
#16701=EDGE_CURVE('',#13492,#13491,#8393,.T.);
#16702=EDGE_CURVE('',#13492,#13493,#2259,.T.);
#16703=EDGE_CURVE('',#13494,#13493,#8394,.T.);
#16704=EDGE_CURVE('',#13494,#13495,#2260,.T.);
#16705=EDGE_CURVE('',#13496,#13495,#8395,.T.);
#16706=EDGE_CURVE('',#13496,#13497,#2261,.T.);
#16707=EDGE_CURVE('',#13490,#13497,#8396,.T.);
#16708=EDGE_CURVE('',#13498,#13499,#2262,.T.);
#16709=EDGE_CURVE('',#13479,#13499,#8397,.T.);
#16710=EDGE_CURVE('',#13478,#13498,#8398,.T.);
#16711=EDGE_CURVE('',#13498,#13500,#2263,.T.);
#16712=EDGE_CURVE('',#13500,#13501,#2264,.T.);
#16713=EDGE_CURVE('',#13499,#13501,#2265,.T.);
#16714=EDGE_CURVE('',#13501,#13502,#8399,.T.);
#16715=EDGE_CURVE('',#13503,#13502,#2266,.T.);
#16716=EDGE_CURVE('',#13499,#13503,#8400,.T.);
#16717=EDGE_CURVE('',#13504,#13505,#2267,.T.);
#16718=EDGE_CURVE('',#13504,#13506,#8401,.T.);
#16719=EDGE_CURVE('',#13507,#13506,#8402,.T.);
#16720=EDGE_CURVE('',#13508,#13507,#2268,.T.);
#16721=EDGE_CURVE('',#13509,#13508,#8403,.T.);
#16722=EDGE_CURVE('',#13509,#13505,#8404,.T.);
#16723=EDGE_CURVE('',#13510,#13510,#2269,.T.);
#16724=EDGE_CURVE('',#13511,#13512,#2270,.T.);
#16725=EDGE_CURVE('',#13511,#13513,#8405,.T.);
#16726=EDGE_CURVE('',#13514,#13513,#8406,.T.);
#16727=EDGE_CURVE('',#13515,#13514,#2271,.T.);
#16728=EDGE_CURVE('',#13516,#13515,#8407,.T.);
#16729=EDGE_CURVE('',#13516,#13512,#8408,.T.);
#16730=EDGE_CURVE('',#13517,#13517,#2272,.T.);
#16731=EDGE_CURVE('',#13518,#13519,#2273,.T.);
#16732=EDGE_CURVE('',#13518,#13502,#8409,.T.);
#16733=EDGE_CURVE('',#13520,#13500,#8410,.T.);
#16734=EDGE_CURVE('',#13520,#13519,#8411,.T.);
#16735=EDGE_CURVE('',#13521,#13521,#2274,.T.);
#16736=EDGE_CURVE('',#13522,#13523,#2275,.T.);
#16737=EDGE_CURVE('',#13522,#13524,#8412,.T.);
#16738=EDGE_CURVE('',#13525,#13524,#8413,.T.);
#16739=EDGE_CURVE('',#13526,#13525,#2276,.T.);
#16740=EDGE_CURVE('',#13527,#13526,#8414,.T.);
#16741=EDGE_CURVE('',#13527,#13523,#8415,.T.);
#16742=EDGE_CURVE('',#13528,#13528,#2277,.T.);
#16743=EDGE_CURVE('',#13486,#13521,#8416,.T.);
#16744=EDGE_CURVE('',#13487,#13517,#8417,.T.);
#16745=EDGE_CURVE('',#13488,#13510,#8418,.T.);
#16746=EDGE_CURVE('',#13489,#13528,#8419,.T.);
#16747=EDGE_CURVE('',#13505,#13529,#2278,.T.);
#16748=EDGE_CURVE('',#13530,#13529,#2279,.T.);
#16749=EDGE_CURVE('',#13504,#13530,#2280,.T.);
#16750=EDGE_CURVE('',#13531,#13530,#743,.T.);
#16751=EDGE_CURVE('',#13532,#13531,#2281,.T.);
#16752=EDGE_CURVE('',#13532,#13504,#744,.T.);
#16753=EDGE_CURVE('',#13533,#13534,#2282,.T.);
#16754=EDGE_CURVE('',#13533,#13535,#8420,.T.);
#16755=EDGE_CURVE('',#13535,#13531,#2283,.T.);
#16756=EDGE_CURVE('',#13529,#13536,#745,.T.);
#16757=EDGE_CURVE('',#13536,#13537,#2284,.T.);
#16758=EDGE_CURVE('',#13537,#13538,#746,.T.);
#16759=EDGE_CURVE('',#13538,#13539,#2285,.T.);
#16760=EDGE_CURVE('',#13539,#13540,#747,.T.);
#16761=EDGE_CURVE('',#13540,#13541,#2286,.T.);
#16762=EDGE_CURVE('',#13541,#13542,#748,.T.);
#16763=EDGE_CURVE('',#13542,#13543,#2287,.T.);
#16764=EDGE_CURVE('',#13543,#13544,#749,.T.);
#16765=EDGE_CURVE('',#13544,#13545,#2288,.T.);
#16766=EDGE_CURVE('',#13545,#13546,#750,.T.);
#16767=EDGE_CURVE('',#13546,#13547,#2289,.T.);
#16768=EDGE_CURVE('',#13547,#13548,#751,.T.);
#16769=EDGE_CURVE('',#13548,#13535,#2290,.T.);
#16770=EDGE_CURVE('',#13534,#13533,#2291,.T.);
#16771=EDGE_CURVE('',#13549,#13550,#2292,.T.);
#16772=EDGE_CURVE('',#13549,#13531,#2293,.T.);
#16773=EDGE_CURVE('',#13550,#13548,#2294,.T.);
#16774=EDGE_CURVE('',#13551,#13550,#8421,.T.);
#16775=EDGE_CURVE('',#13552,#13551,#8422,.T.);
#16776=EDGE_CURVE('',#13549,#13552,#8423,.T.);
#16777=EDGE_CURVE('',#13553,#13554,#2295,.T.);
#16778=EDGE_CURVE('',#13555,#13553,#8424,.T.);
#16779=EDGE_CURVE('',#13556,#13555,#8425,.T.);
#16780=EDGE_CURVE('',#13554,#13556,#8426,.T.);
#16781=EDGE_CURVE('',#13557,#13558,#2296,.T.);
#16782=EDGE_CURVE('',#13559,#13558,#8427,.T.);
#16783=EDGE_CURVE('',#13560,#13559,#8428,.T.);
#16784=EDGE_CURVE('',#13557,#13560,#8429,.T.);
#16785=EDGE_CURVE('',#13561,#13562,#2297,.T.);
#16786=EDGE_CURVE('',#13563,#13561,#8430,.T.);
#16787=EDGE_CURVE('',#13564,#13563,#8431,.T.);
#16788=EDGE_CURVE('',#13562,#13564,#8432,.T.);
#16789=EDGE_CURVE('',#13532,#13549,#2298,.T.);
#16790=EDGE_CURVE('',#13565,#13552,#752,.T.);
#16791=EDGE_CURVE('',#13532,#13565,#8433,.T.);
#16792=EDGE_CURVE('',#13565,#13506,#2299,.T.);
#16793=EDGE_CURVE('',#13566,#13565,#2300,.T.);
#16794=EDGE_CURVE('',#13566,#13506,#2301,.T.);
#16795=EDGE_CURVE('',#13567,#13566,#8434,.T.);
#16796=EDGE_CURVE('',#13567,#13507,#2302,.T.);
#16797=EDGE_CURVE('',#13568,#13567,#2303,.T.);
#16798=EDGE_CURVE('',#13568,#13508,#2304,.T.);
#16799=EDGE_CURVE('',#13483,#13567,#8435,.T.);
#16800=EDGE_CURVE('',#13482,#13568,#8436,.T.);
#16801=EDGE_CURVE('',#13569,#13570,#8437,.T.);
#16802=EDGE_CURVE('',#13570,#13571,#753,.T.);
#16803=EDGE_CURVE('',#13571,#13572,#8438,.T.);
#16804=EDGE_CURVE('',#13572,#13573,#754,.T.);
#16805=EDGE_CURVE('',#13573,#13568,#8439,.T.);
#16806=EDGE_CURVE('',#13481,#13569,#8440,.T.);
#16807=EDGE_CURVE('',#13570,#13513,#2305,.T.);
#16808=EDGE_CURVE('',#13569,#13514,#2306,.T.);
#16809=EDGE_CURVE('',#13574,#13569,#2307,.T.);
#16810=EDGE_CURVE('',#13574,#13515,#2308,.T.);
#16811=EDGE_CURVE('',#13480,#13574,#8441,.T.);
#16812=EDGE_CURVE('',#13575,#13576,#755,.T.);
#16813=EDGE_CURVE('',#13576,#13574,#8442,.T.);
#16814=EDGE_CURVE('',#13503,#13577,#756,.T.);
#16815=EDGE_CURVE('',#13577,#13575,#8443,.T.);
#16816=EDGE_CURVE('',#13559,#13578,#757,.T.);
#16817=EDGE_CURVE('',#13576,#13578,#758,.T.);
#16818=EDGE_CURVE('',#13575,#13559,#2309,.T.);
#16819=EDGE_CURVE('',#13558,#13579,#2310,.T.);
#16820=EDGE_CURVE('',#13578,#13579,#8444,.T.);
#16821=EDGE_CURVE('',#13558,#13540,#2311,.T.);
#16822=EDGE_CURVE('',#13579,#13540,#2312,.T.);
#16823=EDGE_CURVE('',#13512,#13579,#759,.T.);
#16824=EDGE_CURVE('',#13512,#13539,#2313,.T.);
#16825=EDGE_CURVE('',#13516,#13578,#2314,.T.);
#16826=EDGE_CURVE('',#13576,#13516,#2315,.T.);
#16827=EDGE_CURVE('',#13511,#13538,#2316,.T.);
#16828=EDGE_CURVE('',#13580,#13537,#2317,.T.);
#16829=EDGE_CURVE('',#13580,#13511,#760,.T.);
#16830=EDGE_CURVE('',#13580,#13581,#8445,.T.);
#16831=EDGE_CURVE('',#13581,#13513,#2318,.T.);
#16832=EDGE_CURVE('',#13570,#13581,#2319,.T.);
#16833=EDGE_CURVE('',#13581,#13556,#761,.T.);
#16834=EDGE_CURVE('',#13571,#13556,#2320,.T.);
#16835=EDGE_CURVE('',#13572,#13555,#2321,.T.);
#16836=EDGE_CURVE('',#13555,#13582,#762,.T.);
#16837=EDGE_CURVE('',#13573,#13582,#763,.T.);
#16838=EDGE_CURVE('',#13553,#13583,#2322,.T.);
#16839=EDGE_CURVE('',#13582,#13583,#8446,.T.);
#16840=EDGE_CURVE('',#13553,#13536,#2323,.T.);
#16841=EDGE_CURVE('',#13583,#13536,#2324,.T.);
#16842=EDGE_CURVE('',#13505,#13583,#764,.T.);
#16843=EDGE_CURVE('',#13509,#13582,#2325,.T.);
#16844=EDGE_CURVE('',#13573,#13509,#2326,.T.);
#16845=EDGE_CURVE('',#13554,#13537,#2327,.T.);
#16846=EDGE_CURVE('',#13580,#13554,#2328,.T.);
#16847=EDGE_CURVE('',#13557,#13541,#2329,.T.);
#16848=EDGE_CURVE('',#13523,#13584,#765,.T.);
#16849=EDGE_CURVE('',#13584,#13548,#2330,.T.);
#16850=EDGE_CURVE('',#13523,#13547,#2331,.T.);
#16851=EDGE_CURVE('',#13527,#13585,#2332,.T.);
#16852=EDGE_CURVE('',#13585,#13584,#8447,.T.);
#16853=EDGE_CURVE('',#13550,#13584,#2333,.T.);
#16854=EDGE_CURVE('',#13551,#13585,#766,.T.);
#16855=EDGE_CURVE('',#13586,#13585,#767,.T.);
#16856=EDGE_CURVE('',#13587,#13586,#768,.T.);
#16857=EDGE_CURVE('',#13587,#13551,#2334,.T.);
#16858=EDGE_CURVE('',#13588,#13587,#8448,.T.);
#16859=EDGE_CURVE('',#13588,#13552,#2335,.T.);
#16860=EDGE_CURVE('',#13566,#13588,#769,.T.);
#16861=EDGE_CURVE('',#13586,#13589,#8449,.T.);
#16862=EDGE_CURVE('',#13484,#13589,#8450,.T.);
#16863=EDGE_CURVE('',#13589,#13590,#2336,.T.);
#16864=EDGE_CURVE('',#13485,#13590,#8451,.T.);
#16865=EDGE_CURVE('',#13589,#13526,#2337,.T.);
#16866=EDGE_CURVE('',#13590,#13525,#2338,.T.);
#16867=EDGE_CURVE('',#13591,#13524,#2339,.T.);
#16868=EDGE_CURVE('',#13590,#13591,#8452,.T.);
#16869=EDGE_CURVE('',#13591,#13592,#770,.T.);
#16870=EDGE_CURVE('',#13592,#13593,#8453,.T.);
#16871=EDGE_CURVE('',#13593,#13594,#771,.T.);
#16872=EDGE_CURVE('',#13594,#13498,#8454,.T.);
#16873=EDGE_CURVE('',#13594,#13520,#2340,.T.);
#16874=EDGE_CURVE('',#13520,#13595,#2341,.T.);
#16875=EDGE_CURVE('',#13594,#13595,#2342,.T.);
#16876=EDGE_CURVE('',#13519,#13596,#772,.T.);
#16877=EDGE_CURVE('',#13595,#13596,#8455,.T.);
#16878=EDGE_CURVE('',#13596,#13544,#2343,.T.);
#16879=EDGE_CURVE('',#13519,#13543,#2344,.T.);
#16880=EDGE_CURVE('',#13518,#13542,#2345,.T.);
#16881=EDGE_CURVE('',#13597,#13541,#2346,.T.);
#16882=EDGE_CURVE('',#13597,#13518,#773,.T.);
#16883=EDGE_CURVE('',#13597,#13598,#8456,.T.);
#16884=EDGE_CURVE('',#13598,#13502,#2347,.T.);
#16885=EDGE_CURVE('',#13503,#13598,#2348,.T.);
#16886=EDGE_CURVE('',#13598,#13560,#774,.T.);
#16887=EDGE_CURVE('',#13577,#13560,#2349,.T.);
#16888=EDGE_CURVE('',#13597,#13557,#2350,.T.);
#16889=EDGE_CURVE('',#13561,#13596,#2351,.T.);
#16890=EDGE_CURVE('',#13561,#13544,#2352,.T.);
#16891=EDGE_CURVE('',#13563,#13595,#775,.T.);
#16892=EDGE_CURVE('',#13593,#13563,#2353,.T.);
#16893=EDGE_CURVE('',#13592,#13564,#2354,.T.);
#16894=EDGE_CURVE('',#13591,#13599,#2355,.T.);
#16895=EDGE_CURVE('',#13599,#13564,#776,.T.);
#16896=EDGE_CURVE('',#13600,#13562,#2356,.T.);
#16897=EDGE_CURVE('',#13600,#13599,#8457,.T.);
#16898=EDGE_CURVE('',#13600,#13545,#2357,.T.);
#16899=EDGE_CURVE('',#13562,#13545,#2358,.T.);
#16900=EDGE_CURVE('',#13600,#13522,#777,.T.);
#16901=EDGE_CURVE('',#13522,#13546,#2359,.T.);
#16902=EDGE_CURVE('',#13599,#13524,#2360,.T.);
#16903=EDGE_CURVE('',#13586,#13527,#2361,.T.);
#16904=EDGE_CURVE('',#13601,#13601,#2362,.T.);
#16905=EDGE_CURVE('',#13601,#13534,#2363,.T.);
#16906=EDGE_CURVE('',#13602,#13602,#2364,.T.);
#16907=EDGE_CURVE('',#13603,#13604,#2365,.T.);
#16908=EDGE_CURVE('',#13604,#13603,#2366,.T.);
#16909=EDGE_CURVE('',#13604,#13602,#2367,.T.);
#16910=EDGE_CURVE('',#13605,#13605,#2368,.T.);
#16911=EDGE_CURVE('',#13605,#13603,#8458,.T.);
#16912=EDGE_CURVE('',#13606,#13606,#2369,.T.);
#16913=EDGE_CURVE('',#13607,#13607,#2370,.T.);
#16914=EDGE_CURVE('',#13607,#13606,#8459,.T.);
#16915=EDGE_CURVE('',#13608,#13608,#2371,.T.);
#16916=EDGE_CURVE('',#13609,#13609,#2372,.T.);
#16917=EDGE_CURVE('',#13609,#13608,#8460,.T.);
#16918=EDGE_CURVE('',#13610,#13610,#2373,.T.);
#16919=EDGE_CURVE('',#13611,#13611,#2374,.T.);
#16920=EDGE_CURVE('',#13611,#13610,#8461,.T.);
#16921=EDGE_CURVE('',#13612,#13612,#2375,.T.);
#16922=EDGE_CURVE('',#13613,#13613,#2376,.T.);
#16923=EDGE_CURVE('',#13613,#13612,#8462,.T.);
#16924=EDGE_CURVE('',#13614,#13614,#2377,.T.);
#16925=EDGE_CURVE('',#13615,#13615,#2378,.T.);
#16926=EDGE_CURVE('',#13615,#13614,#8463,.T.);
#16927=EDGE_CURVE('',#13616,#13616,#2379,.T.);
#16928=EDGE_CURVE('',#13617,#13617,#2380,.T.);
#16929=EDGE_CURVE('',#13617,#13616,#8464,.T.);
#16930=EDGE_CURVE('',#13618,#13619,#2381,.T.);
#16931=EDGE_CURVE('',#13619,#13620,#8465,.T.);
#16932=EDGE_CURVE('',#13620,#13621,#2382,.T.);
#16933=EDGE_CURVE('',#13621,#13622,#8466,.T.);
#16934=EDGE_CURVE('',#13622,#13623,#2383,.T.);
#16935=EDGE_CURVE('',#13623,#13624,#8467,.T.);
#16936=EDGE_CURVE('',#13624,#13625,#2384,.T.);
#16937=EDGE_CURVE('',#13625,#13618,#8468,.T.);
#16938=EDGE_CURVE('',#13490,#13619,#8469,.T.);
#16939=EDGE_CURVE('',#13491,#13618,#8470,.T.);
#16940=EDGE_CURVE('',#13492,#13625,#8471,.T.);
#16941=EDGE_CURVE('',#13493,#13624,#8472,.T.);
#16942=EDGE_CURVE('',#13494,#13623,#8473,.T.);
#16943=EDGE_CURVE('',#13495,#13622,#8474,.T.);
#16944=EDGE_CURVE('',#13496,#13621,#8475,.T.);
#16945=EDGE_CURVE('',#13497,#13620,#8476,.T.);
#21572=ORIENTED_EDGE('',*,*,#16688,.T.);
#21573=ORIENTED_EDGE('',*,*,#16689,.T.);
#21574=ORIENTED_EDGE('',*,*,#16690,.T.);
#21575=ORIENTED_EDGE('',*,*,#16691,.T.);
#21576=ORIENTED_EDGE('',*,*,#16692,.T.);
#21577=ORIENTED_EDGE('',*,*,#16693,.T.);
#21578=ORIENTED_EDGE('',*,*,#16694,.T.);
#21579=ORIENTED_EDGE('',*,*,#16695,.T.);
#21580=ORIENTED_EDGE('',*,*,#16696,.T.);
#21581=ORIENTED_EDGE('',*,*,#16697,.T.);
#21582=ORIENTED_EDGE('',*,*,#16698,.T.);
#21583=ORIENTED_EDGE('',*,*,#16699,.T.);
#21584=ORIENTED_EDGE('',*,*,#16700,.T.);
#21585=ORIENTED_EDGE('',*,*,#16701,.F.);
#21586=ORIENTED_EDGE('',*,*,#16702,.T.);
#21587=ORIENTED_EDGE('',*,*,#16703,.F.);
#21588=ORIENTED_EDGE('',*,*,#16704,.T.);
#21589=ORIENTED_EDGE('',*,*,#16705,.F.);
#21590=ORIENTED_EDGE('',*,*,#16706,.T.);
#21591=ORIENTED_EDGE('',*,*,#16707,.F.);
#21592=ORIENTED_EDGE('',*,*,#16708,.T.);
#21593=ORIENTED_EDGE('',*,*,#16709,.F.);
#21594=ORIENTED_EDGE('',*,*,#16688,.F.);
#21595=ORIENTED_EDGE('',*,*,#16710,.T.);
#21596=ORIENTED_EDGE('',*,*,#16708,.F.);
#21597=ORIENTED_EDGE('',*,*,#16711,.T.);
#21598=ORIENTED_EDGE('',*,*,#16712,.T.);
#21599=ORIENTED_EDGE('',*,*,#16713,.F.);
#21600=ORIENTED_EDGE('',*,*,#16714,.T.);
#21601=ORIENTED_EDGE('',*,*,#16715,.F.);
#21602=ORIENTED_EDGE('',*,*,#16716,.F.);
#21603=ORIENTED_EDGE('',*,*,#16713,.T.);
#21604=ORIENTED_EDGE('',*,*,#16717,.F.);
#21605=ORIENTED_EDGE('',*,*,#16718,.T.);
#21606=ORIENTED_EDGE('',*,*,#16719,.F.);
#21607=ORIENTED_EDGE('',*,*,#16720,.F.);
#21608=ORIENTED_EDGE('',*,*,#16721,.F.);
#21609=ORIENTED_EDGE('',*,*,#16722,.T.);
#21610=ORIENTED_EDGE('',*,*,#16723,.F.);
#21611=ORIENTED_EDGE('',*,*,#16724,.F.);
#21612=ORIENTED_EDGE('',*,*,#16725,.T.);
#21613=ORIENTED_EDGE('',*,*,#16726,.F.);
#21614=ORIENTED_EDGE('',*,*,#16727,.F.);
#21615=ORIENTED_EDGE('',*,*,#16728,.F.);
#21616=ORIENTED_EDGE('',*,*,#16729,.T.);
#21617=ORIENTED_EDGE('',*,*,#16730,.F.);
#21618=ORIENTED_EDGE('',*,*,#16731,.F.);
#21619=ORIENTED_EDGE('',*,*,#16732,.T.);
#21620=ORIENTED_EDGE('',*,*,#16714,.F.);
#21621=ORIENTED_EDGE('',*,*,#16712,.F.);
#21622=ORIENTED_EDGE('',*,*,#16733,.F.);
#21623=ORIENTED_EDGE('',*,*,#16734,.T.);
#21624=ORIENTED_EDGE('',*,*,#16735,.F.);
#21625=ORIENTED_EDGE('',*,*,#16736,.F.);
#21626=ORIENTED_EDGE('',*,*,#16737,.T.);
#21627=ORIENTED_EDGE('',*,*,#16738,.F.);
#21628=ORIENTED_EDGE('',*,*,#16739,.F.);
#21629=ORIENTED_EDGE('',*,*,#16740,.F.);
#21630=ORIENTED_EDGE('',*,*,#16741,.T.);
#21631=ORIENTED_EDGE('',*,*,#16742,.F.);
#21632=ORIENTED_EDGE('',*,*,#16696,.F.);
#21633=ORIENTED_EDGE('',*,*,#16743,.T.);
#21634=ORIENTED_EDGE('',*,*,#16735,.T.);
#21635=ORIENTED_EDGE('',*,*,#16743,.F.);
#21636=ORIENTED_EDGE('',*,*,#16697,.F.);
#21637=ORIENTED_EDGE('',*,*,#16744,.T.);
#21638=ORIENTED_EDGE('',*,*,#16730,.T.);
#21639=ORIENTED_EDGE('',*,*,#16744,.F.);
#21640=ORIENTED_EDGE('',*,*,#16698,.F.);
#21641=ORIENTED_EDGE('',*,*,#16745,.T.);
#21642=ORIENTED_EDGE('',*,*,#16723,.T.);
#21643=ORIENTED_EDGE('',*,*,#16745,.F.);
#21644=ORIENTED_EDGE('',*,*,#16699,.F.);
#21645=ORIENTED_EDGE('',*,*,#16746,.T.);
#21646=ORIENTED_EDGE('',*,*,#16742,.T.);
#21647=ORIENTED_EDGE('',*,*,#16746,.F.);
#21648=ORIENTED_EDGE('',*,*,#16717,.T.);
#21649=ORIENTED_EDGE('',*,*,#16747,.T.);
#21650=ORIENTED_EDGE('',*,*,#16748,.F.);
#21651=ORIENTED_EDGE('',*,*,#16749,.F.);
#21652=ORIENTED_EDGE('',*,*,#16750,.F.);
#21653=ORIENTED_EDGE('',*,*,#16751,.F.);
#21654=ORIENTED_EDGE('',*,*,#16752,.T.);
#21655=ORIENTED_EDGE('',*,*,#16749,.T.);
#21656=ORIENTED_EDGE('',*,*,#16753,.F.);
#21657=ORIENTED_EDGE('',*,*,#16754,.T.);
#21658=ORIENTED_EDGE('',*,*,#16755,.T.);
#21659=ORIENTED_EDGE('',*,*,#16750,.T.);
#21660=ORIENTED_EDGE('',*,*,#16748,.T.);
#21661=ORIENTED_EDGE('',*,*,#16756,.T.);
#21662=ORIENTED_EDGE('',*,*,#16757,.T.);
#21663=ORIENTED_EDGE('',*,*,#16758,.T.);
#21664=ORIENTED_EDGE('',*,*,#16759,.T.);
#21665=ORIENTED_EDGE('',*,*,#16760,.T.);
#21666=ORIENTED_EDGE('',*,*,#16761,.T.);
#21667=ORIENTED_EDGE('',*,*,#16762,.T.);
#21668=ORIENTED_EDGE('',*,*,#16763,.T.);
#21669=ORIENTED_EDGE('',*,*,#16764,.T.);
#21670=ORIENTED_EDGE('',*,*,#16765,.T.);
#21671=ORIENTED_EDGE('',*,*,#16766,.T.);
#21672=ORIENTED_EDGE('',*,*,#16767,.T.);
#21673=ORIENTED_EDGE('',*,*,#16768,.T.);
#21674=ORIENTED_EDGE('',*,*,#16769,.T.);
#21675=ORIENTED_EDGE('',*,*,#16754,.F.);
#21676=ORIENTED_EDGE('',*,*,#16770,.F.);
#21677=ORIENTED_EDGE('',*,*,#16771,.F.);
#21678=ORIENTED_EDGE('',*,*,#16772,.T.);
#21679=ORIENTED_EDGE('',*,*,#16755,.F.);
#21680=ORIENTED_EDGE('',*,*,#16769,.F.);
#21681=ORIENTED_EDGE('',*,*,#16773,.F.);
#21682=ORIENTED_EDGE('',*,*,#16771,.T.);
#21683=ORIENTED_EDGE('',*,*,#16774,.F.);
#21684=ORIENTED_EDGE('',*,*,#16775,.F.);
#21685=ORIENTED_EDGE('',*,*,#16776,.F.);
#21686=ORIENTED_EDGE('',*,*,#16777,.F.);
#21687=ORIENTED_EDGE('',*,*,#16778,.F.);
#21688=ORIENTED_EDGE('',*,*,#16779,.F.);
#21689=ORIENTED_EDGE('',*,*,#16780,.F.);
#21690=ORIENTED_EDGE('',*,*,#16781,.T.);
#21691=ORIENTED_EDGE('',*,*,#16782,.F.);
#21692=ORIENTED_EDGE('',*,*,#16783,.F.);
#21693=ORIENTED_EDGE('',*,*,#16784,.F.);
#21694=ORIENTED_EDGE('',*,*,#16785,.F.);
#21695=ORIENTED_EDGE('',*,*,#16786,.F.);
#21696=ORIENTED_EDGE('',*,*,#16787,.F.);
#21697=ORIENTED_EDGE('',*,*,#16788,.F.);
#21698=ORIENTED_EDGE('',*,*,#16789,.T.);
#21699=ORIENTED_EDGE('',*,*,#16776,.T.);
#21700=ORIENTED_EDGE('',*,*,#16790,.F.);
#21701=ORIENTED_EDGE('',*,*,#16791,.F.);
#21702=ORIENTED_EDGE('',*,*,#16789,.F.);
#21703=ORIENTED_EDGE('',*,*,#16751,.T.);
#21704=ORIENTED_EDGE('',*,*,#16772,.F.);
#21705=ORIENTED_EDGE('',*,*,#16752,.F.);
#21706=ORIENTED_EDGE('',*,*,#16791,.T.);
#21707=ORIENTED_EDGE('',*,*,#16792,.T.);
#21708=ORIENTED_EDGE('',*,*,#16718,.F.);
#21709=ORIENTED_EDGE('',*,*,#16792,.F.);
#21710=ORIENTED_EDGE('',*,*,#16793,.F.);
#21711=ORIENTED_EDGE('',*,*,#16794,.T.);
#21712=ORIENTED_EDGE('',*,*,#16719,.T.);
#21713=ORIENTED_EDGE('',*,*,#16794,.F.);
#21714=ORIENTED_EDGE('',*,*,#16795,.F.);
#21715=ORIENTED_EDGE('',*,*,#16796,.T.);
#21716=ORIENTED_EDGE('',*,*,#16797,.F.);
#21717=ORIENTED_EDGE('',*,*,#16798,.T.);
#21718=ORIENTED_EDGE('',*,*,#16720,.T.);
#21719=ORIENTED_EDGE('',*,*,#16796,.F.);
#21720=ORIENTED_EDGE('',*,*,#16797,.T.);
#21721=ORIENTED_EDGE('',*,*,#16799,.F.);
#21722=ORIENTED_EDGE('',*,*,#16692,.F.);
#21723=ORIENTED_EDGE('',*,*,#16800,.T.);
#21724=ORIENTED_EDGE('',*,*,#16801,.T.);
#21725=ORIENTED_EDGE('',*,*,#16802,.T.);
#21726=ORIENTED_EDGE('',*,*,#16803,.T.);
#21727=ORIENTED_EDGE('',*,*,#16804,.T.);
#21728=ORIENTED_EDGE('',*,*,#16805,.T.);
#21729=ORIENTED_EDGE('',*,*,#16800,.F.);
#21730=ORIENTED_EDGE('',*,*,#16691,.F.);
#21731=ORIENTED_EDGE('',*,*,#16806,.T.);
#21732=ORIENTED_EDGE('',*,*,#16726,.T.);
#21733=ORIENTED_EDGE('',*,*,#16807,.F.);
#21734=ORIENTED_EDGE('',*,*,#16801,.F.);
#21735=ORIENTED_EDGE('',*,*,#16808,.T.);
#21736=ORIENTED_EDGE('',*,*,#16809,.F.);
#21737=ORIENTED_EDGE('',*,*,#16810,.T.);
#21738=ORIENTED_EDGE('',*,*,#16727,.T.);
#21739=ORIENTED_EDGE('',*,*,#16808,.F.);
#21740=ORIENTED_EDGE('',*,*,#16809,.T.);
#21741=ORIENTED_EDGE('',*,*,#16806,.F.);
#21742=ORIENTED_EDGE('',*,*,#16690,.F.);
#21743=ORIENTED_EDGE('',*,*,#16811,.T.);
#21744=ORIENTED_EDGE('',*,*,#16812,.T.);
#21745=ORIENTED_EDGE('',*,*,#16813,.T.);
#21746=ORIENTED_EDGE('',*,*,#16811,.F.);
#21747=ORIENTED_EDGE('',*,*,#16689,.F.);
#21748=ORIENTED_EDGE('',*,*,#16709,.T.);
#21749=ORIENTED_EDGE('',*,*,#16716,.T.);
#21750=ORIENTED_EDGE('',*,*,#16814,.T.);
#21751=ORIENTED_EDGE('',*,*,#16815,.T.);
#21752=ORIENTED_EDGE('',*,*,#16816,.T.);
#21753=ORIENTED_EDGE('',*,*,#16817,.F.);
#21754=ORIENTED_EDGE('',*,*,#16812,.F.);
#21755=ORIENTED_EDGE('',*,*,#16818,.T.);
#21756=ORIENTED_EDGE('',*,*,#16819,.T.);
#21757=ORIENTED_EDGE('',*,*,#16820,.F.);
#21758=ORIENTED_EDGE('',*,*,#16816,.F.);
#21759=ORIENTED_EDGE('',*,*,#16782,.T.);
#21760=ORIENTED_EDGE('',*,*,#16819,.F.);
#21761=ORIENTED_EDGE('',*,*,#16821,.T.);
#21762=ORIENTED_EDGE('',*,*,#16822,.F.);
#21763=ORIENTED_EDGE('',*,*,#16823,.T.);
#21764=ORIENTED_EDGE('',*,*,#16822,.T.);
#21765=ORIENTED_EDGE('',*,*,#16760,.F.);
#21766=ORIENTED_EDGE('',*,*,#16824,.F.);
#21767=ORIENTED_EDGE('',*,*,#16823,.F.);
#21768=ORIENTED_EDGE('',*,*,#16729,.F.);
#21769=ORIENTED_EDGE('',*,*,#16825,.T.);
#21770=ORIENTED_EDGE('',*,*,#16820,.T.);
#21771=ORIENTED_EDGE('',*,*,#16825,.F.);
#21772=ORIENTED_EDGE('',*,*,#16826,.F.);
#21773=ORIENTED_EDGE('',*,*,#16817,.T.);
#21774=ORIENTED_EDGE('',*,*,#16813,.F.);
#21775=ORIENTED_EDGE('',*,*,#16826,.T.);
#21776=ORIENTED_EDGE('',*,*,#16728,.T.);
#21777=ORIENTED_EDGE('',*,*,#16810,.F.);
#21778=ORIENTED_EDGE('',*,*,#16724,.T.);
#21779=ORIENTED_EDGE('',*,*,#16824,.T.);
#21780=ORIENTED_EDGE('',*,*,#16759,.F.);
#21781=ORIENTED_EDGE('',*,*,#16827,.F.);
#21782=ORIENTED_EDGE('',*,*,#16758,.F.);
#21783=ORIENTED_EDGE('',*,*,#16828,.F.);
#21784=ORIENTED_EDGE('',*,*,#16829,.T.);
#21785=ORIENTED_EDGE('',*,*,#16827,.T.);
#21786=ORIENTED_EDGE('',*,*,#16829,.F.);
#21787=ORIENTED_EDGE('',*,*,#16830,.T.);
#21788=ORIENTED_EDGE('',*,*,#16831,.T.);
#21789=ORIENTED_EDGE('',*,*,#16725,.F.);
#21790=ORIENTED_EDGE('',*,*,#16831,.F.);
#21791=ORIENTED_EDGE('',*,*,#16832,.F.);
#21792=ORIENTED_EDGE('',*,*,#16807,.T.);
#21793=ORIENTED_EDGE('',*,*,#16802,.F.);
#21794=ORIENTED_EDGE('',*,*,#16832,.T.);
#21795=ORIENTED_EDGE('',*,*,#16833,.T.);
#21796=ORIENTED_EDGE('',*,*,#16834,.F.);
#21797=ORIENTED_EDGE('',*,*,#16803,.F.);
#21798=ORIENTED_EDGE('',*,*,#16834,.T.);
#21799=ORIENTED_EDGE('',*,*,#16779,.T.);
#21800=ORIENTED_EDGE('',*,*,#16835,.F.);
#21801=ORIENTED_EDGE('',*,*,#16836,.T.);
#21802=ORIENTED_EDGE('',*,*,#16837,.F.);
#21803=ORIENTED_EDGE('',*,*,#16804,.F.);
#21804=ORIENTED_EDGE('',*,*,#16835,.T.);
#21805=ORIENTED_EDGE('',*,*,#16838,.T.);
#21806=ORIENTED_EDGE('',*,*,#16839,.F.);
#21807=ORIENTED_EDGE('',*,*,#16836,.F.);
#21808=ORIENTED_EDGE('',*,*,#16778,.T.);
#21809=ORIENTED_EDGE('',*,*,#16838,.F.);
#21810=ORIENTED_EDGE('',*,*,#16840,.T.);
#21811=ORIENTED_EDGE('',*,*,#16841,.F.);
#21812=ORIENTED_EDGE('',*,*,#16842,.T.);
#21813=ORIENTED_EDGE('',*,*,#16841,.T.);
#21814=ORIENTED_EDGE('',*,*,#16756,.F.);
#21815=ORIENTED_EDGE('',*,*,#16747,.F.);
#21816=ORIENTED_EDGE('',*,*,#16842,.F.);
#21817=ORIENTED_EDGE('',*,*,#16722,.F.);
#21818=ORIENTED_EDGE('',*,*,#16843,.T.);
#21819=ORIENTED_EDGE('',*,*,#16839,.T.);
#21820=ORIENTED_EDGE('',*,*,#16843,.F.);
#21821=ORIENTED_EDGE('',*,*,#16844,.F.);
#21822=ORIENTED_EDGE('',*,*,#16837,.T.);
#21823=ORIENTED_EDGE('',*,*,#16805,.F.);
#21824=ORIENTED_EDGE('',*,*,#16844,.T.);
#21825=ORIENTED_EDGE('',*,*,#16721,.T.);
#21826=ORIENTED_EDGE('',*,*,#16798,.F.);
#21827=ORIENTED_EDGE('',*,*,#16777,.T.);
#21828=ORIENTED_EDGE('',*,*,#16845,.T.);
#21829=ORIENTED_EDGE('',*,*,#16757,.F.);
#21830=ORIENTED_EDGE('',*,*,#16840,.F.);
#21831=ORIENTED_EDGE('',*,*,#16846,.F.);
#21832=ORIENTED_EDGE('',*,*,#16828,.T.);
#21833=ORIENTED_EDGE('',*,*,#16845,.F.);
#21834=ORIENTED_EDGE('',*,*,#16846,.T.);
#21835=ORIENTED_EDGE('',*,*,#16780,.T.);
#21836=ORIENTED_EDGE('',*,*,#16833,.F.);
#21837=ORIENTED_EDGE('',*,*,#16830,.F.);
#21838=ORIENTED_EDGE('',*,*,#16781,.F.);
#21839=ORIENTED_EDGE('',*,*,#16847,.T.);
#21840=ORIENTED_EDGE('',*,*,#16761,.F.);
#21841=ORIENTED_EDGE('',*,*,#16821,.F.);
#21842=ORIENTED_EDGE('',*,*,#16848,.T.);
#21843=ORIENTED_EDGE('',*,*,#16849,.T.);
#21844=ORIENTED_EDGE('',*,*,#16768,.F.);
#21845=ORIENTED_EDGE('',*,*,#16850,.F.);
#21846=ORIENTED_EDGE('',*,*,#16848,.F.);
#21847=ORIENTED_EDGE('',*,*,#16741,.F.);
#21848=ORIENTED_EDGE('',*,*,#16851,.T.);
#21849=ORIENTED_EDGE('',*,*,#16852,.T.);
#21850=ORIENTED_EDGE('',*,*,#16853,.T.);
#21851=ORIENTED_EDGE('',*,*,#16852,.F.);
#21852=ORIENTED_EDGE('',*,*,#16854,.F.);
#21853=ORIENTED_EDGE('',*,*,#16774,.T.);
#21854=ORIENTED_EDGE('',*,*,#16853,.F.);
#21855=ORIENTED_EDGE('',*,*,#16773,.T.);
#21856=ORIENTED_EDGE('',*,*,#16849,.F.);
#21857=ORIENTED_EDGE('',*,*,#16854,.T.);
#21858=ORIENTED_EDGE('',*,*,#16855,.F.);
#21859=ORIENTED_EDGE('',*,*,#16856,.F.);
#21860=ORIENTED_EDGE('',*,*,#16857,.T.);
#21861=ORIENTED_EDGE('',*,*,#16858,.F.);
#21862=ORIENTED_EDGE('',*,*,#16859,.T.);
#21863=ORIENTED_EDGE('',*,*,#16775,.T.);
#21864=ORIENTED_EDGE('',*,*,#16857,.F.);
#21865=ORIENTED_EDGE('',*,*,#16795,.T.);
#21866=ORIENTED_EDGE('',*,*,#16860,.T.);
#21867=ORIENTED_EDGE('',*,*,#16858,.T.);
#21868=ORIENTED_EDGE('',*,*,#16856,.T.);
#21869=ORIENTED_EDGE('',*,*,#16861,.T.);
#21870=ORIENTED_EDGE('',*,*,#16862,.F.);
#21871=ORIENTED_EDGE('',*,*,#16693,.F.);
#21872=ORIENTED_EDGE('',*,*,#16799,.T.);
#21873=ORIENTED_EDGE('',*,*,#16863,.T.);
#21874=ORIENTED_EDGE('',*,*,#16864,.F.);
#21875=ORIENTED_EDGE('',*,*,#16694,.F.);
#21876=ORIENTED_EDGE('',*,*,#16862,.T.);
#21877=ORIENTED_EDGE('',*,*,#16863,.F.);
#21878=ORIENTED_EDGE('',*,*,#16865,.T.);
#21879=ORIENTED_EDGE('',*,*,#16739,.T.);
#21880=ORIENTED_EDGE('',*,*,#16866,.F.);
#21881=ORIENTED_EDGE('',*,*,#16738,.T.);
#21882=ORIENTED_EDGE('',*,*,#16867,.F.);
#21883=ORIENTED_EDGE('',*,*,#16868,.F.);
#21884=ORIENTED_EDGE('',*,*,#16866,.T.);
#21885=ORIENTED_EDGE('',*,*,#16868,.T.);
#21886=ORIENTED_EDGE('',*,*,#16869,.T.);
#21887=ORIENTED_EDGE('',*,*,#16870,.T.);
#21888=ORIENTED_EDGE('',*,*,#16871,.T.);
#21889=ORIENTED_EDGE('',*,*,#16872,.T.);
#21890=ORIENTED_EDGE('',*,*,#16710,.F.);
#21891=ORIENTED_EDGE('',*,*,#16695,.F.);
#21892=ORIENTED_EDGE('',*,*,#16864,.T.);
#21893=ORIENTED_EDGE('',*,*,#16872,.F.);
#21894=ORIENTED_EDGE('',*,*,#16873,.T.);
#21895=ORIENTED_EDGE('',*,*,#16733,.T.);
#21896=ORIENTED_EDGE('',*,*,#16711,.F.);
#21897=ORIENTED_EDGE('',*,*,#16874,.F.);
#21898=ORIENTED_EDGE('',*,*,#16873,.F.);
#21899=ORIENTED_EDGE('',*,*,#16875,.T.);
#21900=ORIENTED_EDGE('',*,*,#16876,.F.);
#21901=ORIENTED_EDGE('',*,*,#16734,.F.);
#21902=ORIENTED_EDGE('',*,*,#16874,.T.);
#21903=ORIENTED_EDGE('',*,*,#16877,.T.);
#21904=ORIENTED_EDGE('',*,*,#16876,.T.);
#21905=ORIENTED_EDGE('',*,*,#16878,.T.);
#21906=ORIENTED_EDGE('',*,*,#16764,.F.);
#21907=ORIENTED_EDGE('',*,*,#16879,.F.);
#21908=ORIENTED_EDGE('',*,*,#16731,.T.);
#21909=ORIENTED_EDGE('',*,*,#16879,.T.);
#21910=ORIENTED_EDGE('',*,*,#16763,.F.);
#21911=ORIENTED_EDGE('',*,*,#16880,.F.);
#21912=ORIENTED_EDGE('',*,*,#16762,.F.);
#21913=ORIENTED_EDGE('',*,*,#16881,.F.);
#21914=ORIENTED_EDGE('',*,*,#16882,.T.);
#21915=ORIENTED_EDGE('',*,*,#16880,.T.);
#21916=ORIENTED_EDGE('',*,*,#16882,.F.);
#21917=ORIENTED_EDGE('',*,*,#16883,.T.);
#21918=ORIENTED_EDGE('',*,*,#16884,.T.);
#21919=ORIENTED_EDGE('',*,*,#16732,.F.);
#21920=ORIENTED_EDGE('',*,*,#16884,.F.);
#21921=ORIENTED_EDGE('',*,*,#16885,.F.);
#21922=ORIENTED_EDGE('',*,*,#16715,.T.);
#21923=ORIENTED_EDGE('',*,*,#16814,.F.);
#21924=ORIENTED_EDGE('',*,*,#16885,.T.);
#21925=ORIENTED_EDGE('',*,*,#16886,.T.);
#21926=ORIENTED_EDGE('',*,*,#16887,.F.);
#21927=ORIENTED_EDGE('',*,*,#16815,.F.);
#21928=ORIENTED_EDGE('',*,*,#16887,.T.);
#21929=ORIENTED_EDGE('',*,*,#16783,.T.);
#21930=ORIENTED_EDGE('',*,*,#16818,.F.);
#21931=ORIENTED_EDGE('',*,*,#16888,.T.);
#21932=ORIENTED_EDGE('',*,*,#16784,.T.);
#21933=ORIENTED_EDGE('',*,*,#16886,.F.);
#21934=ORIENTED_EDGE('',*,*,#16883,.F.);
#21935=ORIENTED_EDGE('',*,*,#16888,.F.);
#21936=ORIENTED_EDGE('',*,*,#16881,.T.);
#21937=ORIENTED_EDGE('',*,*,#16847,.F.);
#21938=ORIENTED_EDGE('',*,*,#16889,.F.);
#21939=ORIENTED_EDGE('',*,*,#16890,.T.);
#21940=ORIENTED_EDGE('',*,*,#16878,.F.);
#21941=ORIENTED_EDGE('',*,*,#16889,.T.);
#21942=ORIENTED_EDGE('',*,*,#16877,.F.);
#21943=ORIENTED_EDGE('',*,*,#16891,.F.);
#21944=ORIENTED_EDGE('',*,*,#16786,.T.);
#21945=ORIENTED_EDGE('',*,*,#16891,.T.);
#21946=ORIENTED_EDGE('',*,*,#16875,.F.);
#21947=ORIENTED_EDGE('',*,*,#16871,.F.);
#21948=ORIENTED_EDGE('',*,*,#16892,.T.);
#21949=ORIENTED_EDGE('',*,*,#16870,.F.);
#21950=ORIENTED_EDGE('',*,*,#16893,.T.);
#21951=ORIENTED_EDGE('',*,*,#16787,.T.);
#21952=ORIENTED_EDGE('',*,*,#16892,.F.);
#21953=ORIENTED_EDGE('',*,*,#16869,.F.);
#21954=ORIENTED_EDGE('',*,*,#16894,.T.);
#21955=ORIENTED_EDGE('',*,*,#16895,.T.);
#21956=ORIENTED_EDGE('',*,*,#16893,.F.);
#21957=ORIENTED_EDGE('',*,*,#16896,.T.);
#21958=ORIENTED_EDGE('',*,*,#16788,.T.);
#21959=ORIENTED_EDGE('',*,*,#16895,.F.);
#21960=ORIENTED_EDGE('',*,*,#16897,.F.);
#21961=ORIENTED_EDGE('',*,*,#16896,.F.);
#21962=ORIENTED_EDGE('',*,*,#16898,.T.);
#21963=ORIENTED_EDGE('',*,*,#16899,.F.);
#21964=ORIENTED_EDGE('',*,*,#16765,.F.);
#21965=ORIENTED_EDGE('',*,*,#16890,.F.);
#21966=ORIENTED_EDGE('',*,*,#16785,.T.);
#21967=ORIENTED_EDGE('',*,*,#16899,.T.);
#21968=ORIENTED_EDGE('',*,*,#16766,.F.);
#21969=ORIENTED_EDGE('',*,*,#16898,.F.);
#21970=ORIENTED_EDGE('',*,*,#16900,.T.);
#21971=ORIENTED_EDGE('',*,*,#16901,.T.);
#21972=ORIENTED_EDGE('',*,*,#16736,.T.);
#21973=ORIENTED_EDGE('',*,*,#16850,.T.);
#21974=ORIENTED_EDGE('',*,*,#16767,.F.);
#21975=ORIENTED_EDGE('',*,*,#16901,.F.);
#21976=ORIENTED_EDGE('',*,*,#16900,.F.);
#21977=ORIENTED_EDGE('',*,*,#16897,.T.);
#21978=ORIENTED_EDGE('',*,*,#16902,.T.);
#21979=ORIENTED_EDGE('',*,*,#16737,.F.);
#21980=ORIENTED_EDGE('',*,*,#16902,.F.);
#21981=ORIENTED_EDGE('',*,*,#16894,.F.);
#21982=ORIENTED_EDGE('',*,*,#16867,.T.);
#21983=ORIENTED_EDGE('',*,*,#16861,.F.);
#21984=ORIENTED_EDGE('',*,*,#16903,.T.);
#21985=ORIENTED_EDGE('',*,*,#16740,.T.);
#21986=ORIENTED_EDGE('',*,*,#16865,.F.);
#21987=ORIENTED_EDGE('',*,*,#16851,.F.);
#21988=ORIENTED_EDGE('',*,*,#16903,.F.);
#21989=ORIENTED_EDGE('',*,*,#16855,.T.);
#21990=ORIENTED_EDGE('',*,*,#16860,.F.);
#21991=ORIENTED_EDGE('',*,*,#16793,.T.);
#21992=ORIENTED_EDGE('',*,*,#16790,.T.);
#21993=ORIENTED_EDGE('',*,*,#16859,.F.);
#21994=ORIENTED_EDGE('',*,*,#16904,.F.);
#21995=ORIENTED_EDGE('',*,*,#16905,.T.);
#21996=ORIENTED_EDGE('',*,*,#16770,.T.);
#21997=ORIENTED_EDGE('',*,*,#16753,.T.);
#21998=ORIENTED_EDGE('',*,*,#16905,.F.);
#21999=ORIENTED_EDGE('',*,*,#16904,.T.);
#22000=ORIENTED_EDGE('',*,*,#16906,.T.);
#22001=ORIENTED_EDGE('',*,*,#16907,.F.);
#22002=ORIENTED_EDGE('',*,*,#16908,.F.);
#22003=ORIENTED_EDGE('',*,*,#16909,.T.);
#22004=ORIENTED_EDGE('',*,*,#16906,.F.);
#22005=ORIENTED_EDGE('',*,*,#16909,.F.);
#22006=ORIENTED_EDGE('',*,*,#16910,.T.);
#22007=ORIENTED_EDGE('',*,*,#16911,.T.);
#22008=ORIENTED_EDGE('',*,*,#16907,.T.);
#22009=ORIENTED_EDGE('',*,*,#16908,.T.);
#22010=ORIENTED_EDGE('',*,*,#16911,.F.);
#22011=ORIENTED_EDGE('',*,*,#16910,.F.);
#22012=ORIENTED_EDGE('',*,*,#16912,.T.);
#22013=ORIENTED_EDGE('',*,*,#16913,.T.);
#22014=ORIENTED_EDGE('',*,*,#16914,.T.);
#22015=ORIENTED_EDGE('',*,*,#16912,.F.);
#22016=ORIENTED_EDGE('',*,*,#16914,.F.);
#22017=ORIENTED_EDGE('',*,*,#16913,.F.);
#22018=ORIENTED_EDGE('',*,*,#16915,.T.);
#22019=ORIENTED_EDGE('',*,*,#16916,.T.);
#22020=ORIENTED_EDGE('',*,*,#16917,.T.);
#22021=ORIENTED_EDGE('',*,*,#16915,.F.);
#22022=ORIENTED_EDGE('',*,*,#16917,.F.);
#22023=ORIENTED_EDGE('',*,*,#16916,.F.);
#22024=ORIENTED_EDGE('',*,*,#16918,.T.);
#22025=ORIENTED_EDGE('',*,*,#16919,.T.);
#22026=ORIENTED_EDGE('',*,*,#16920,.T.);
#22027=ORIENTED_EDGE('',*,*,#16918,.F.);
#22028=ORIENTED_EDGE('',*,*,#16920,.F.);
#22029=ORIENTED_EDGE('',*,*,#16921,.T.);
#22030=ORIENTED_EDGE('',*,*,#16919,.F.);
#22031=ORIENTED_EDGE('',*,*,#16922,.T.);
#22032=ORIENTED_EDGE('',*,*,#16923,.T.);
#22033=ORIENTED_EDGE('',*,*,#16921,.F.);
#22034=ORIENTED_EDGE('',*,*,#16923,.F.);
#22035=ORIENTED_EDGE('',*,*,#16924,.T.);
#22036=ORIENTED_EDGE('',*,*,#16922,.F.);
#22037=ORIENTED_EDGE('',*,*,#16925,.T.);
#22038=ORIENTED_EDGE('',*,*,#16926,.T.);
#22039=ORIENTED_EDGE('',*,*,#16924,.F.);
#22040=ORIENTED_EDGE('',*,*,#16926,.F.);
#22041=ORIENTED_EDGE('',*,*,#16927,.T.);
#22042=ORIENTED_EDGE('',*,*,#16925,.F.);
#22043=ORIENTED_EDGE('',*,*,#16928,.F.);
#22044=ORIENTED_EDGE('',*,*,#16929,.T.);
#22045=ORIENTED_EDGE('',*,*,#16927,.F.);
#22046=ORIENTED_EDGE('',*,*,#16929,.F.);
#22047=ORIENTED_EDGE('',*,*,#16930,.T.);
#22048=ORIENTED_EDGE('',*,*,#16931,.T.);
#22049=ORIENTED_EDGE('',*,*,#16932,.T.);
#22050=ORIENTED_EDGE('',*,*,#16933,.T.);
#22051=ORIENTED_EDGE('',*,*,#16934,.T.);
#22052=ORIENTED_EDGE('',*,*,#16935,.T.);
#22053=ORIENTED_EDGE('',*,*,#16936,.T.);
#22054=ORIENTED_EDGE('',*,*,#16937,.T.);
#22055=ORIENTED_EDGE('',*,*,#16928,.T.);
#22056=ORIENTED_EDGE('',*,*,#16700,.F.);
#22057=ORIENTED_EDGE('',*,*,#16938,.T.);
#22058=ORIENTED_EDGE('',*,*,#16930,.F.);
#22059=ORIENTED_EDGE('',*,*,#16939,.F.);
#22060=ORIENTED_EDGE('',*,*,#16701,.T.);
#22061=ORIENTED_EDGE('',*,*,#16939,.T.);
#22062=ORIENTED_EDGE('',*,*,#16937,.F.);
#22063=ORIENTED_EDGE('',*,*,#16940,.F.);
#22064=ORIENTED_EDGE('',*,*,#16702,.F.);
#22065=ORIENTED_EDGE('',*,*,#16940,.T.);
#22066=ORIENTED_EDGE('',*,*,#16936,.F.);
#22067=ORIENTED_EDGE('',*,*,#16941,.F.);
#22068=ORIENTED_EDGE('',*,*,#16703,.T.);
#22069=ORIENTED_EDGE('',*,*,#16941,.T.);
#22070=ORIENTED_EDGE('',*,*,#16935,.F.);
#22071=ORIENTED_EDGE('',*,*,#16942,.F.);
#22072=ORIENTED_EDGE('',*,*,#16704,.F.);
#22073=ORIENTED_EDGE('',*,*,#16942,.T.);
#22074=ORIENTED_EDGE('',*,*,#16934,.F.);
#22075=ORIENTED_EDGE('',*,*,#16943,.F.);
#22076=ORIENTED_EDGE('',*,*,#16705,.T.);
#22077=ORIENTED_EDGE('',*,*,#16943,.T.);
#22078=ORIENTED_EDGE('',*,*,#16933,.F.);
#22079=ORIENTED_EDGE('',*,*,#16944,.F.);
#22080=ORIENTED_EDGE('',*,*,#16706,.F.);
#22081=ORIENTED_EDGE('',*,*,#16944,.T.);
#22082=ORIENTED_EDGE('',*,*,#16932,.F.);
#22083=ORIENTED_EDGE('',*,*,#16945,.F.);
#22084=ORIENTED_EDGE('',*,*,#16707,.T.);
#22085=ORIENTED_EDGE('',*,*,#16945,.T.);
#22086=ORIENTED_EDGE('',*,*,#16931,.F.);
#22087=ORIENTED_EDGE('',*,*,#16938,.F.);
#31126=PLANE('',#34154);
#31127=PLANE('',#34175);
#31128=PLANE('',#34179);
#31129=PLANE('',#34183);
#31130=PLANE('',#34186);
#31131=PLANE('',#34214);
#31132=PLANE('',#34215);
#31133=PLANE('',#34217);
#31134=PLANE('',#34219);
#31135=PLANE('',#34235);
#31136=PLANE('',#34243);
#31137=PLANE('',#34293);
#31138=PLANE('',#34301);
#31139=PLANE('',#34347);
#31140=PLANE('',#34355);
#31141=PLANE('',#34359);
#31142=PLANE('',#34363);
#31143=PLANE('',#34367);
#31144=PLANE('',#34371);
#31145=PLANE('',#34375);
#31146=PLANE('',#34379);
#31147=PLANE('',#34385);
#31148=PLANE('',#34387);
#31149=PLANE('',#34389);
#31150=PLANE('',#34391);
#31934=ADVANCED_FACE('',(#4253,#1880,#1881,#1882,#1883,#1884),#31126,.F.);
#31935=ADVANCED_FACE('',(#4254),#1045,.T.);
#31936=ADVANCED_FACE('',(#4255),#874,.T.);
#31937=ADVANCED_FACE('',(#4256),#1046,.T.);
#31938=ADVANCED_FACE('',(#4257,#1885),#31127,.T.);
#31939=ADVANCED_FACE('',(#4258,#1886),#31128,.T.);
#31940=ADVANCED_FACE('',(#4259,#1887),#31129,.T.);
#31941=ADVANCED_FACE('',(#4260,#1888),#31130,.T.);
#31942=ADVANCED_FACE('',(#4261),#1047,.F.);
#31943=ADVANCED_FACE('',(#4262),#1048,.F.);
#31944=ADVANCED_FACE('',(#4263),#1049,.F.);
#31945=ADVANCED_FACE('',(#4264),#1050,.F.);
#31946=ADVANCED_FACE('',(#4265),#875,.F.);
#31947=ADVANCED_FACE('',(#4266),#854,.F.);
#31948=ADVANCED_FACE('',(#4267),#1051,.T.);
#31949=ADVANCED_FACE('',(#4268),#876,.F.);
#31950=ADVANCED_FACE('',(#4269),#31131,.T.);
#31951=ADVANCED_FACE('',(#4270),#31132,.T.);
#31952=ADVANCED_FACE('',(#4271),#31133,.T.);
#31953=ADVANCED_FACE('',(#4272),#31134,.T.);
#31954=ADVANCED_FACE('',(#4273),#1052,.F.);
#31955=ADVANCED_FACE('',(#4274),#710,.F.);
#31956=ADVANCED_FACE('',(#4275),#1053,.T.);
#31957=ADVANCED_FACE('',(#4276),#711,.T.);
#31958=ADVANCED_FACE('',(#4277),#1054,.T.);
#31959=ADVANCED_FACE('',(#4278),#877,.T.);
#31960=ADVANCED_FACE('',(#4279),#1055,.T.);
#31961=ADVANCED_FACE('',(#4280),#31135,.T.);
#31962=ADVANCED_FACE('',(#4281),#1056,.T.);
#31963=ADVANCED_FACE('',(#4282),#878,.T.);
#31964=ADVANCED_FACE('',(#4283),#1057,.T.);
#31965=ADVANCED_FACE('',(#4284),#31136,.T.);
#31966=ADVANCED_FACE('',(#4285),#855,.T.);
#31967=ADVANCED_FACE('',(#4286),#1058,.F.);
#31968=ADVANCED_FACE('',(#4287),#712,.F.);
#31969=ADVANCED_FACE('',(#4288),#856,.F.);
#31970=ADVANCED_FACE('',(#4289),#1059,.T.);
#31971=ADVANCED_FACE('',(#4290),#713,.T.);
#31972=ADVANCED_FACE('',(#4291),#1060,.T.);
#31973=ADVANCED_FACE('',(#4292),#879,.F.);
#31974=ADVANCED_FACE('',(#4293),#857,.F.);
#31975=ADVANCED_FACE('',(#4294),#1061,.T.);
#31976=ADVANCED_FACE('',(#4295),#714,.T.);
#31977=ADVANCED_FACE('',(#4296),#858,.T.);
#31978=ADVANCED_FACE('',(#4297),#1062,.T.);
#31979=ADVANCED_FACE('',(#4298),#859,.T.);
#31980=ADVANCED_FACE('',(#4299),#1063,.F.);
#31981=ADVANCED_FACE('',(#4300),#715,.F.);
#31982=ADVANCED_FACE('',(#4301),#860,.F.);
#31983=ADVANCED_FACE('',(#4302),#1064,.T.);
#31984=ADVANCED_FACE('',(#4303),#716,.T.);
#31985=ADVANCED_FACE('',(#4304),#1065,.T.);
#31986=ADVANCED_FACE('',(#4305),#880,.F.);
#31987=ADVANCED_FACE('',(#4306),#717,.F.);
#31988=ADVANCED_FACE('',(#4307),#1066,.F.);
#31989=ADVANCED_FACE('',(#4308),#881,.F.);
#31990=ADVANCED_FACE('',(#4309),#861,.F.);
#31991=ADVANCED_FACE('',(#4310),#1067,.T.);
#31992=ADVANCED_FACE('',(#4311),#1068,.F.);
#31993=ADVANCED_FACE('',(#4312),#718,.F.);
#31994=ADVANCED_FACE('',(#4313),#862,.T.);
#31995=ADVANCED_FACE('',(#4314),#1069,.T.);
#31996=ADVANCED_FACE('',(#4315),#31137,.T.);
#31997=ADVANCED_FACE('',(#4316),#1070,.T.);
#31998=ADVANCED_FACE('',(#4317),#882,.T.);
#31999=ADVANCED_FACE('',(#4318),#1071,.T.);
#32000=ADVANCED_FACE('',(#4319),#31138,.T.);
#32001=ADVANCED_FACE('',(#4320),#1072,.T.);
#32002=ADVANCED_FACE('',(#4321),#719,.T.);
#32003=ADVANCED_FACE('',(#4322),#1073,.T.);
#32004=ADVANCED_FACE('',(#4323),#863,.F.);
#32005=ADVANCED_FACE('',(#4324),#883,.F.);
#32006=ADVANCED_FACE('',(#4325),#864,.F.);
#32007=ADVANCED_FACE('',(#4326),#1074,.T.);
#32008=ADVANCED_FACE('',(#4327),#720,.T.);
#32009=ADVANCED_FACE('',(#4328),#865,.T.);
#32010=ADVANCED_FACE('',(#4329),#1075,.T.);
#32011=ADVANCED_FACE('',(#4330),#1076,.F.);
#32012=ADVANCED_FACE('',(#4331),#721,.F.);
#32013=ADVANCED_FACE('',(#4332),#722,.F.);
#32014=ADVANCED_FACE('',(#4333),#1077,.F.);
#32015=ADVANCED_FACE('',(#4334),#866,.T.);
#32016=ADVANCED_FACE('',(#4335),#1078,.T.);
#32017=ADVANCED_FACE('',(#4336),#867,.T.);
#32018=ADVANCED_FACE('',(#4337),#1079,.F.);
#32019=ADVANCED_FACE('',(#4338),#723,.F.);
#32020=ADVANCED_FACE('',(#4339),#884,.F.);
#32021=ADVANCED_FACE('',(#4340),#868,.F.);
#32022=ADVANCED_FACE('',(#4341),#885,.F.);
#32023=ADVANCED_FACE('',(#4342),#1080,.T.);
#32024=ADVANCED_FACE('',(#4343),#724,.T.);
#32025=ADVANCED_FACE('',(#4344),#1081,.T.);
#32026=ADVANCED_FACE('',(#4345),#725,.T.);
#32027=ADVANCED_FACE('',(#4346),#869,.T.);
#32028=ADVANCED_FACE('',(#4347),#886,.T.);
#32029=ADVANCED_FACE('',(#4348,#1889),#31139,.T.);
#32030=ADVANCED_FACE('',(#4349),#887,.T.);
#32031=ADVANCED_FACE('',(#4350),#1082,.T.);
#32032=ADVANCED_FACE('',(#4351,#1890),#31140,.T.);
#32033=ADVANCED_FACE('',(#4352),#1083,.F.);
#32034=ADVANCED_FACE('',(#4353,#1891),#31141,.T.);
#32035=ADVANCED_FACE('',(#4354),#1084,.T.);
#32036=ADVANCED_FACE('',(#4355,#1892),#31142,.T.);
#32037=ADVANCED_FACE('',(#4356),#1085,.F.);
#32038=ADVANCED_FACE('',(#4357,#1893),#31143,.F.);
#32039=ADVANCED_FACE('',(#4358),#1086,.T.);
#32040=ADVANCED_FACE('',(#4359,#1894),#31144,.F.);
#32041=ADVANCED_FACE('',(#4360),#1087,.F.);
#32042=ADVANCED_FACE('',(#4361,#1895),#31145,.F.);
#32043=ADVANCED_FACE('',(#4362),#1088,.F.);
#32044=ADVANCED_FACE('',(#4363,#1896),#31146,.T.);
#32045=ADVANCED_FACE('',(#4364),#1089,.T.);
#32046=ADVANCED_FACE('',(#4365),#31147,.F.);
#32047=ADVANCED_FACE('',(#4366),#1090,.T.);
#32048=ADVANCED_FACE('',(#4367),#31148,.F.);
#32049=ADVANCED_FACE('',(#4368),#1091,.T.);
#32050=ADVANCED_FACE('',(#4369),#31149,.F.);
#32051=ADVANCED_FACE('',(#4370),#1092,.T.);
#32052=ADVANCED_FACE('',(#4371),#31150,.F.);
#33792=CLOSED_SHELL('',(#31934,#31935,#31936,#31937,#31938,#31939,#31940,
#31941,#31942,#31943,#31944,#31945,#31946,#31947,#31948,#31949,#31950,#31951,
#31952,#31953,#31954,#31955,#31956,#31957,#31958,#31959,#31960,#31961,#31962,
#31963,#31964,#31965,#31966,#31967,#31968,#31969,#31970,#31971,#31972,#31973,
#31974,#31975,#31976,#31977,#31978,#31979,#31980,#31981,#31982,#31983,#31984,
#31985,#31986,#31987,#31988,#31989,#31990,#31991,#31992,#31993,#31994,#31995,
#31996,#31997,#31998,#31999,#32000,#32001,#32002,#32003,#32004,#32005,#32006,
#32007,#32008,#32009,#32010,#32011,#32012,#32013,#32014,#32015,#32016,#32017,
#32018,#32019,#32020,#32021,#32022,#32023,#32024,#32025,#32026,#32027,#32028,
#32029,#32030,#32031,#32032,#32033,#32034,#32035,#32036,#32037,#32038,#32039,
#32040,#32041,#32042,#32043,#32044,#32045,#32046,#32047,#32048,#32049,#32050,
#32051,#32052));
#34153=AXIS2_PLACEMENT_3D('',#48955,#38291,#38292);
#34154=AXIS2_PLACEMENT_3D('',#48956,#38293,#38294);
#34155=AXIS2_PLACEMENT_3D('',#48959,#38295,#38296);
#34156=AXIS2_PLACEMENT_3D('',#48963,#38298,#38299);
#34157=AXIS2_PLACEMENT_3D('',#48967,#38301,#38302);
#34158=AXIS2_PLACEMENT_3D('',#48971,#38304,#38305);
#34159=AXIS2_PLACEMENT_3D('',#48974,#38307,#38308);
#34160=AXIS2_PLACEMENT_3D('',#48976,#38309,#38310);
#34161=AXIS2_PLACEMENT_3D('',#48978,#38311,#38312);
#34162=AXIS2_PLACEMENT_3D('',#48980,#38313,#38314);
#34163=AXIS2_PLACEMENT_3D('',#48983,#38315,#38316);
#34164=AXIS2_PLACEMENT_3D('',#48987,#38318,#38319);
#34165=AXIS2_PLACEMENT_3D('',#48991,#38321,#38322);
#34166=AXIS2_PLACEMENT_3D('',#48995,#38324,#38325);
#34167=AXIS2_PLACEMENT_3D('',#48997,#38327,#38328);
#34168=AXIS2_PLACEMENT_3D('',#49000,#38329,#38330);
#34169=AXIS2_PLACEMENT_3D('',#49003,#38333,#38334);
#34170=AXIS2_PLACEMENT_3D('',#49005,#38335,#38336);
#34171=AXIS2_PLACEMENT_3D('',#49007,#38337,#38338);
#34172=AXIS2_PLACEMENT_3D('',#49008,#38339,#38340);
#34173=AXIS2_PLACEMENT_3D('',#49009,#38341,#38342);
#34174=AXIS2_PLACEMENT_3D('',#49013,#38344,#38345);
#34175=AXIS2_PLACEMENT_3D('',#49015,#38347,#38348);
#34176=AXIS2_PLACEMENT_3D('',#49018,#38349,#38350);
#34177=AXIS2_PLACEMENT_3D('',#49024,#38353,#38354);
#34178=AXIS2_PLACEMENT_3D('',#49029,#38357,#38358);
#34179=AXIS2_PLACEMENT_3D('',#49030,#38359,#38360);
#34180=AXIS2_PLACEMENT_3D('',#49033,#38361,#38362);
#34181=AXIS2_PLACEMENT_3D('',#49039,#38365,#38366);
#34182=AXIS2_PLACEMENT_3D('',#49044,#38369,#38370);
#34183=AXIS2_PLACEMENT_3D('',#49045,#38371,#38372);
#34184=AXIS2_PLACEMENT_3D('',#49048,#38373,#38374);
#34185=AXIS2_PLACEMENT_3D('',#49054,#38378,#38379);
#34186=AXIS2_PLACEMENT_3D('',#49055,#38380,#38381);
#34187=AXIS2_PLACEMENT_3D('',#49058,#38382,#38383);
#34188=AXIS2_PLACEMENT_3D('',#49064,#38386,#38387);
#34189=AXIS2_PLACEMENT_3D('',#49069,#38390,#38391);
#34190=AXIS2_PLACEMENT_3D('',#49070,#38392,#38393);
#34191=AXIS2_PLACEMENT_3D('',#49072,#38395,#38396);
#34192=AXIS2_PLACEMENT_3D('',#49074,#38398,#38399);
#34193=AXIS2_PLACEMENT_3D('',#49076,#38401,#38402);
#34194=AXIS2_PLACEMENT_3D('',#49078,#38404,#38405);
#34195=AXIS2_PLACEMENT_3D('',#49080,#38406,#38407);
#34196=AXIS2_PLACEMENT_3D('',#49082,#38408,#38409);
#34197=AXIS2_PLACEMENT_3D('',#49083,#38410,#38411);
#34198=AXIS2_PLACEMENT_3D('',#49131,#38412,#38413);
#34199=AXIS2_PLACEMENT_3D('',#49154,#38414,#38415);
#34200=AXIS2_PLACEMENT_3D('',#49157,#38416,#38417);
#34201=AXIS2_PLACEMENT_3D('',#49160,#38419,#38420);
#34202=AXIS2_PLACEMENT_3D('',#49172,#38421,#38422);
#34203=AXIS2_PLACEMENT_3D('',#49184,#38423,#38424);
#34204=AXIS2_PLACEMENT_3D('',#49196,#38425,#38426);
#34205=AXIS2_PLACEMENT_3D('',#49208,#38427,#38428);
#34206=AXIS2_PLACEMENT_3D('',#49220,#38429,#38430);
#34207=AXIS2_PLACEMENT_3D('',#49232,#38431,#38432);
#34208=AXIS2_PLACEMENT_3D('',#49243,#38433,#38434);
#34209=AXIS2_PLACEMENT_3D('',#49244,#38435,#38436);
#34210=AXIS2_PLACEMENT_3D('',#49245,#38437,#38438);
#34211=AXIS2_PLACEMENT_3D('',#49248,#38439,#38440);
#34212=AXIS2_PLACEMENT_3D('',#49249,#38441,#38442);
#34213=AXIS2_PLACEMENT_3D('',#49250,#38443,#38444);
#34214=AXIS2_PLACEMENT_3D('',#49251,#38445,#38446);
#34215=AXIS2_PLACEMENT_3D('',#49257,#38450,#38451);
#34216=AXIS2_PLACEMENT_3D('',#49260,#38452,#38453);
#34217=AXIS2_PLACEMENT_3D('',#49266,#38457,#38458);
#34218=AXIS2_PLACEMENT_3D('',#49269,#38459,#38460);
#34219=AXIS2_PLACEMENT_3D('',#49275,#38464,#38465);
#34220=AXIS2_PLACEMENT_3D('',#49278,#38466,#38467);
#34221=AXIS2_PLACEMENT_3D('',#49284,#38471,#38472);
#34222=AXIS2_PLACEMENT_3D('',#49285,#38473,#38474);
#34223=AXIS2_PLACEMENT_3D('',#49343,#38476,#38477);
#34224=AXIS2_PLACEMENT_3D('',#49344,#38478,#38479);
#34225=AXIS2_PLACEMENT_3D('',#49345,#38480,#38481);
#34226=AXIS2_PLACEMENT_3D('',#49346,#38482,#38483);
#34227=AXIS2_PLACEMENT_3D('',#49348,#38484,#38485);
#34228=AXIS2_PLACEMENT_3D('',#49349,#38486,#38487);
#34229=AXIS2_PLACEMENT_3D('',#49350,#38488,#38489);
#34230=AXIS2_PLACEMENT_3D('',#49353,#38491,#38492);
#34231=AXIS2_PLACEMENT_3D('',#49354,#38493,#38494);
#34232=AXIS2_PLACEMENT_3D('',#49356,#38495,#38496);
#34233=AXIS2_PLACEMENT_3D('',#49357,#38497,#38498);
#34234=AXIS2_PLACEMENT_3D('',#49358,#38499,#38500);
#34235=AXIS2_PLACEMENT_3D('',#49361,#38503,#38504);
#34236=AXIS2_PLACEMENT_3D('',#49391,#38509,#38510);
#34237=AXIS2_PLACEMENT_3D('',#49392,#38511,#38512);
#34238=AXIS2_PLACEMENT_3D('',#49393,#38513,#38514);
#34239=AXIS2_PLACEMENT_3D('',#49394,#38515,#38516);
#34240=AXIS2_PLACEMENT_3D('',#49396,#38517,#38518);
#34241=AXIS2_PLACEMENT_3D('',#49397,#38519,#38520);
#34242=AXIS2_PLACEMENT_3D('',#49398,#38521,#38522);
#34243=AXIS2_PLACEMENT_3D('',#49400,#38524,#38525);
#34244=AXIS2_PLACEMENT_3D('',#49578,#38528,#38529);
#34245=AXIS2_PLACEMENT_3D('',#49579,#38530,#38531);
#34246=AXIS2_PLACEMENT_3D('',#49581,#38532,#38533);
#34247=AXIS2_PLACEMENT_3D('',#49583,#38535,#38536);
#34248=AXIS2_PLACEMENT_3D('',#49584,#38537,#38538);
#34249=AXIS2_PLACEMENT_3D('',#49585,#38539,#38540);
#34250=AXIS2_PLACEMENT_3D('',#49644,#38541,#38542);
#34251=AXIS2_PLACEMENT_3D('',#49645,#38543,#38544);
#34252=AXIS2_PLACEMENT_3D('',#49646,#38545,#38546);
#34253=AXIS2_PLACEMENT_3D('',#49647,#38547,#38548);
#34254=AXIS2_PLACEMENT_3D('',#49648,#38549,#38550);
#34255=AXIS2_PLACEMENT_3D('',#49649,#38551,#38552);
#34256=AXIS2_PLACEMENT_3D('',#49650,#38553,#38554);
#34257=AXIS2_PLACEMENT_3D('',#49651,#38555,#38556);
#34258=AXIS2_PLACEMENT_3D('',#49689,#38557,#38558);
#34259=AXIS2_PLACEMENT_3D('',#49699,#38559,#38560);
#34260=AXIS2_PLACEMENT_3D('',#49702,#38562,#38563);
#34261=AXIS2_PLACEMENT_3D('',#49703,#38564,#38565);
#34262=AXIS2_PLACEMENT_3D('',#49704,#38566,#38567);
#34263=AXIS2_PLACEMENT_3D('',#49813,#38568,#38569);
#34264=AXIS2_PLACEMENT_3D('',#49814,#38570,#38571);
#34265=AXIS2_PLACEMENT_3D('',#49815,#38572,#38573);
#34266=AXIS2_PLACEMENT_3D('',#49968,#38574,#38575);
#34267=AXIS2_PLACEMENT_3D('',#49970,#38576,#38577);
#34268=AXIS2_PLACEMENT_3D('',#49972,#38579,#38580);
#34269=AXIS2_PLACEMENT_3D('',#49973,#38581,#38582);
#34270=AXIS2_PLACEMENT_3D('',#49974,#38583,#38584);
#34271=AXIS2_PLACEMENT_3D('',#50020,#38585,#38586);
#34272=AXIS2_PLACEMENT_3D('',#50021,#38587,#38588);
#34273=AXIS2_PLACEMENT_3D('',#50022,#38589,#38590);
#34274=AXIS2_PLACEMENT_3D('',#50023,#38591,#38592);
#34275=AXIS2_PLACEMENT_3D('',#50024,#38593,#38594);
#34276=AXIS2_PLACEMENT_3D('',#50025,#38595,#38596);
#34277=AXIS2_PLACEMENT_3D('',#50026,#38597,#38598);
#34278=AXIS2_PLACEMENT_3D('',#50027,#38599,#38600);
#34279=AXIS2_PLACEMENT_3D('',#50028,#38601,#38602);
#34280=AXIS2_PLACEMENT_3D('',#50029,#38603,#38604);
#34281=AXIS2_PLACEMENT_3D('',#50030,#38605,#38606);
#34282=AXIS2_PLACEMENT_3D('',#50031,#38607,#38608);
#34283=AXIS2_PLACEMENT_3D('',#50091,#38609,#38610);
#34284=AXIS2_PLACEMENT_3D('',#50092,#38611,#38612);
#34285=AXIS2_PLACEMENT_3D('',#50093,#38613,#38614);
#34286=AXIS2_PLACEMENT_3D('',#50095,#38615,#38616);
#34287=AXIS2_PLACEMENT_3D('',#50097,#38618,#38619);
#34288=AXIS2_PLACEMENT_3D('',#50098,#38620,#38621);
#34289=AXIS2_PLACEMENT_3D('',#50154,#38622,#38623);
#34290=AXIS2_PLACEMENT_3D('',#50254,#38624,#38625);
#34291=AXIS2_PLACEMENT_3D('',#50255,#38626,#38627);
#34292=AXIS2_PLACEMENT_3D('',#50258,#38629,#38630);
#34293=AXIS2_PLACEMENT_3D('',#50259,#38631,#38632);
#34294=AXIS2_PLACEMENT_3D('',#50273,#38635,#38636);
#34295=AXIS2_PLACEMENT_3D('',#50275,#38637,#38638);
#34296=AXIS2_PLACEMENT_3D('',#50277,#38640,#38641);
#34297=AXIS2_PLACEMENT_3D('',#50278,#38642,#38643);
#34298=AXIS2_PLACEMENT_3D('',#50279,#38644,#38645);
#34299=AXIS2_PLACEMENT_3D('',#50280,#38646,#38647);
#34300=AXIS2_PLACEMENT_3D('',#50282,#38648,#38649);
#34301=AXIS2_PLACEMENT_3D('',#50284,#38651,#38652);
#34302=AXIS2_PLACEMENT_3D('',#50310,#38655,#38656);
#34303=AXIS2_PLACEMENT_3D('',#50311,#38657,#38658);
#34304=AXIS2_PLACEMENT_3D('',#50312,#38659,#38660);
#34305=AXIS2_PLACEMENT_3D('',#50314,#38661,#38662);
#34306=AXIS2_PLACEMENT_3D('',#50315,#38663,#38664);
#34307=AXIS2_PLACEMENT_3D('',#50316,#38665,#38666);
#34308=AXIS2_PLACEMENT_3D('',#50364,#38668,#38669);
#34309=AXIS2_PLACEMENT_3D('',#50365,#38670,#38671);
#34310=AXIS2_PLACEMENT_3D('',#50366,#38672,#38673);
#34311=AXIS2_PLACEMENT_3D('',#50367,#38674,#38675);
#34312=AXIS2_PLACEMENT_3D('',#50405,#38676,#38677);
#34313=AXIS2_PLACEMENT_3D('',#50428,#38678,#38679);
#34314=AXIS2_PLACEMENT_3D('',#50431,#38681,#38682);
#34315=AXIS2_PLACEMENT_3D('',#50432,#38683,#38684);
#34316=AXIS2_PLACEMENT_3D('',#50433,#38685,#38686);
#34317=AXIS2_PLACEMENT_3D('',#50542,#38687,#38688);
#34318=AXIS2_PLACEMENT_3D('',#50543,#38689,#38690);
#34319=AXIS2_PLACEMENT_3D('',#50544,#38691,#38692);
#34320=AXIS2_PLACEMENT_3D('',#50545,#38693,#38694);
#34321=AXIS2_PLACEMENT_3D('',#50546,#38695,#38696);
#34322=AXIS2_PLACEMENT_3D('',#50547,#38697,#38698);
#34323=AXIS2_PLACEMENT_3D('',#50548,#38699,#38700);
#34324=AXIS2_PLACEMENT_3D('',#50549,#38701,#38702);
#34325=AXIS2_PLACEMENT_3D('',#50550,#38703,#38704);
#34326=AXIS2_PLACEMENT_3D('',#50650,#38705,#38706);
#34327=AXIS2_PLACEMENT_3D('',#50651,#38707,#38708);
#34328=AXIS2_PLACEMENT_3D('',#50652,#38709,#38710);
#34329=AXIS2_PLACEMENT_3D('',#50698,#38711,#38712);
#34330=AXIS2_PLACEMENT_3D('',#50763,#38713,#38714);
#34331=AXIS2_PLACEMENT_3D('',#50765,#38715,#38716);
#34332=AXIS2_PLACEMENT_3D('',#50767,#38718,#38719);
#34333=AXIS2_PLACEMENT_3D('',#50768,#38720,#38721);
#34334=AXIS2_PLACEMENT_3D('',#50769,#38722,#38723);
#34335=AXIS2_PLACEMENT_3D('',#50770,#38724,#38725);
#34336=AXIS2_PLACEMENT_3D('',#50816,#38726,#38727);
#34337=AXIS2_PLACEMENT_3D('',#50817,#38728,#38729);
#34338=AXIS2_PLACEMENT_3D('',#50818,#38730,#38731);
#34339=AXIS2_PLACEMENT_3D('',#50819,#38732,#38733);
#34340=AXIS2_PLACEMENT_3D('',#50820,#38734,#38735);
#34341=AXIS2_PLACEMENT_3D('',#50821,#38736,#38737);
#34342=AXIS2_PLACEMENT_3D('',#50822,#38738,#38739);
#34343=AXIS2_PLACEMENT_3D('',#50823,#38740,#38741);
#34344=AXIS2_PLACEMENT_3D('',#50868,#38742,#38743);
#34345=AXIS2_PLACEMENT_3D('',#50870,#38744,#38745);
#34346=AXIS2_PLACEMENT_3D('',#50871,#38746,#38747);
#34347=AXIS2_PLACEMENT_3D('',#50872,#38748,#38749);
#34348=AXIS2_PLACEMENT_3D('',#50874,#38750,#38751);
#34349=AXIS2_PLACEMENT_3D('',#50875,#38752,#38753);
#34350=AXIS2_PLACEMENT_3D('',#50878,#38754,#38755);
#34351=AXIS2_PLACEMENT_3D('',#50879,#38756,#38757);
#34352=AXIS2_PLACEMENT_3D('',#50880,#38758,#38759);
#34353=AXIS2_PLACEMENT_3D('',#50881,#38760,#38761);
#34354=AXIS2_PLACEMENT_3D('',#50883,#38762,#38763);
#34355=AXIS2_PLACEMENT_3D('',#50885,#38765,#38766);
#34356=AXIS2_PLACEMENT_3D('',#50887,#38767,#38768);
#34357=AXIS2_PLACEMENT_3D('',#50888,#38769,#38770);
#34358=AXIS2_PLACEMENT_3D('',#50890,#38771,#38772);
#34359=AXIS2_PLACEMENT_3D('',#50892,#38774,#38775);
#34360=AXIS2_PLACEMENT_3D('',#50894,#38776,#38777);
#34361=AXIS2_PLACEMENT_3D('',#50895,#38778,#38779);
#34362=AXIS2_PLACEMENT_3D('',#50897,#38780,#38781);
#34363=AXIS2_PLACEMENT_3D('',#50899,#38783,#38784);
#34364=AXIS2_PLACEMENT_3D('',#50901,#38785,#38786);
#34365=AXIS2_PLACEMENT_3D('',#50902,#38787,#38788);
#34366=AXIS2_PLACEMENT_3D('',#50904,#38789,#38790);
#34367=AXIS2_PLACEMENT_3D('',#50906,#38792,#38793);
#34368=AXIS2_PLACEMENT_3D('',#50908,#38794,#38795);
#34369=AXIS2_PLACEMENT_3D('',#50909,#38796,#38797);
#34370=AXIS2_PLACEMENT_3D('',#50911,#38798,#38799);
#34371=AXIS2_PLACEMENT_3D('',#50913,#38801,#38802);
#34372=AXIS2_PLACEMENT_3D('',#50915,#38803,#38804);
#34373=AXIS2_PLACEMENT_3D('',#50916,#38805,#38806);
#34374=AXIS2_PLACEMENT_3D('',#50918,#38807,#38808);
#34375=AXIS2_PLACEMENT_3D('',#50920,#38810,#38811);
#34376=AXIS2_PLACEMENT_3D('',#50922,#38812,#38813);
#34377=AXIS2_PLACEMENT_3D('',#50923,#38814,#38815);
#34378=AXIS2_PLACEMENT_3D('',#50925,#38816,#38817);
#34379=AXIS2_PLACEMENT_3D('',#50927,#38819,#38820);
#34380=AXIS2_PLACEMENT_3D('',#50930,#38821,#38822);
#34381=AXIS2_PLACEMENT_3D('',#50934,#38824,#38825);
#34382=AXIS2_PLACEMENT_3D('',#50938,#38827,#38828);
#34383=AXIS2_PLACEMENT_3D('',#50942,#38830,#38831);
#34384=AXIS2_PLACEMENT_3D('',#50944,#38833,#38834);
#34385=AXIS2_PLACEMENT_3D('',#50947,#38837,#38838);
#34386=AXIS2_PLACEMENT_3D('',#50949,#38840,#38841);
#34387=AXIS2_PLACEMENT_3D('',#50951,#38843,#38844);
#34388=AXIS2_PLACEMENT_3D('',#50953,#38846,#38847);
#34389=AXIS2_PLACEMENT_3D('',#50955,#38849,#38850);
#34390=AXIS2_PLACEMENT_3D('',#50957,#38852,#38853);
#34391=AXIS2_PLACEMENT_3D('',#50959,#38855,#38856);
#38291=DIRECTION('axis',(0.,0.,1.));
#38292=DIRECTION('refdir',(1.,0.,0.));
#38293=DIRECTION('center_axis',(5.00596043934461E-16,1.,1.12027918221652E-15));
#38294=DIRECTION('ref_axis',(1.,-5.00596043934455E-16,-5.57179392097267E-15));
#38295=DIRECTION('center_axis',(-5.00596043934461E-16,-1.,-1.12027918221652E-15));
#38296=DIRECTION('ref_axis',(-1.,5.00596043934455E-16,5.57179392097267E-15));
#38297=DIRECTION('',(1.,-5.00596043934455E-16,-5.57179392097267E-15));
#38298=DIRECTION('center_axis',(-5.00596043934461E-16,-1.,-1.12027918221652E-15));
#38299=DIRECTION('ref_axis',(-5.57179392097266E-15,1.12027918221652E-15,
-1.));
#38300=DIRECTION('',(5.57179392097266E-15,-1.12027918221652E-15,1.));
#38301=DIRECTION('center_axis',(-5.00596043934461E-16,-1.,-1.12027918221652E-15));
#38302=DIRECTION('ref_axis',(1.,-5.00596043934455E-16,-5.57179392097267E-15));
#38303=DIRECTION('',(-1.,5.00596043934455E-16,5.57179392097267E-15));
#38304=DIRECTION('center_axis',(-5.00596043934461E-16,-1.,-1.12027918221652E-15));
#38305=DIRECTION('ref_axis',(5.57179392097266E-15,-1.12027918221652E-15,
1.));
#38306=DIRECTION('',(-5.57179392097266E-15,1.12027918221652E-15,-1.));
#38307=DIRECTION('center_axis',(5.00596043934461E-16,1.,1.12027918221652E-15));
#38308=DIRECTION('ref_axis',(1.,-5.00596043934455E-16,-5.57179392097267E-15));
#38309=DIRECTION('center_axis',(5.00596043934461E-16,1.,1.12027918221652E-15));
#38310=DIRECTION('ref_axis',(1.,-5.00596043934455E-16,-5.57179392097267E-15));
#38311=DIRECTION('center_axis',(5.00596043934461E-16,1.,1.12027918221652E-15));
#38312=DIRECTION('ref_axis',(1.,-5.00596043934455E-16,-5.57179392097267E-15));
#38313=DIRECTION('center_axis',(5.00596043934461E-16,1.,1.12027918221652E-15));
#38314=DIRECTION('ref_axis',(1.,-5.00596043934455E-16,-5.57179392097267E-15));
#38315=DIRECTION('center_axis',(-5.00596043934461E-16,-1.,-1.12027918221652E-15));
#38316=DIRECTION('ref_axis',(5.57179392097266E-15,-1.12027918221652E-15,
1.));
#38317=DIRECTION('',(1.,-5.00596043934455E-16,-5.57179392097266E-15));
#38318=DIRECTION('center_axis',(-5.00596043934461E-16,-1.,-1.12027918221652E-15));
#38319=DIRECTION('ref_axis',(1.,-5.00596043934455E-16,-5.57179392097267E-15));
#38320=DIRECTION('',(-5.57179392097266E-15,1.12027918221652E-15,-1.));
#38321=DIRECTION('center_axis',(-5.00596043934461E-16,-1.,-1.12027918221652E-15));
#38322=DIRECTION('ref_axis',(-5.57179392097266E-15,1.12027918221652E-15,
-1.));
#38323=DIRECTION('',(-1.,5.00596043934455E-16,5.57179392097266E-15));
#38324=DIRECTION('center_axis',(-5.00596043934461E-16,-1.,-1.12027918221652E-15));
#38325=DIRECTION('ref_axis',(-1.,5.00596043934455E-16,5.57179392097267E-15));
#38326=DIRECTION('',(5.57179392097266E-15,-1.12027918221652E-15,1.));
#38327=DIRECTION('center_axis',(5.00596043934461E-16,1.,1.12027918221652E-15));
#38328=DIRECTION('ref_axis',(1.,-5.00596043934455E-16,-5.57179392097267E-15));
#38329=DIRECTION('center_axis',(-5.00596043934461E-16,-1.,-1.12027918221652E-15));
#38330=DIRECTION('ref_axis',(-1.,5.00596043934455E-16,5.57179392097267E-15));
#38331=DIRECTION('',(5.14815917377939E-11,1.,1.12027918192968E-15));
#38332=DIRECTION('',(5.00596044180201E-16,1.,4.41054475357122E-11));
#38333=DIRECTION('center_axis',(5.00596043934461E-16,1.,1.12027918221652E-15));
#38334=DIRECTION('ref_axis',(-0.999766740157022,0.,0.0215978071989372));
#38335=DIRECTION('center_axis',(2.79269661923508E-9,1.12027918081851E-15,
-1.));
#38336=DIRECTION('ref_axis',(-1.,5.00596047063061E-16,-2.79269661923508E-9));
#38337=DIRECTION('center_axis',(-5.00596043934461E-16,-1.,-1.12027918221652E-15));
#38338=DIRECTION('ref_axis',(-1.,5.00596043934455E-16,5.57179392097267E-15));
#38339=DIRECTION('center_axis',(1.,-5.00596043934455E-16,-5.57179392097267E-15));
#38340=DIRECTION('ref_axis',(-5.57179392097266E-15,1.12027918221652E-15,
-1.));
#38341=DIRECTION('center_axis',(1.,-5.00596043934455E-16,-5.57179392097267E-15));
#38342=DIRECTION('ref_axis',(-5.57179392097266E-15,1.12027918221652E-15,
-1.));
#38343=DIRECTION('',(1.,-5.00596043934455E-16,-5.57179392097267E-15));
#38344=DIRECTION('center_axis',(1.,-5.00596043934455E-16,-5.57179392097267E-15));
#38345=DIRECTION('ref_axis',(-5.57179392097266E-15,1.12027918221652E-15,
-1.));
#38346=DIRECTION('',(0.999999999999992,-1.07234894352195E-7,7.46977803037953E-8));
#38347=DIRECTION('center_axis',(5.00596043934461E-16,1.,1.12027918221652E-15));
#38348=DIRECTION('ref_axis',(1.,-5.00596043934455E-16,-5.57179392097267E-15));
#38349=DIRECTION('center_axis',(5.00596043934461E-16,1.,1.12027918221652E-15));
#38350=DIRECTION('ref_axis',(0.560028488394602,-1.20846949316291E-15,0.828473350317593));
#38351=DIRECTION('',(0.626626299212589,1.16622759427748E-9,0.779319883703178));
#38352=DIRECTION('',(-1.,5.00596043934455E-16,5.57179392097267E-15));
#38353=DIRECTION('center_axis',(-5.00596043934461E-16,-1.,-1.12027918221652E-15));
#38354=DIRECTION('ref_axis',(1.,-5.00596043934455E-16,-5.57179392097267E-15));
#38355=DIRECTION('',(5.57179392097267E-15,-1.12027918221652E-15,1.));
#38356=DIRECTION('',(-0.779319883703586,-1.08364385785013E-9,-0.626626299212081));
#38357=DIRECTION('center_axis',(5.00596043934461E-16,1.,1.12027918221652E-15));
#38358=DIRECTION('ref_axis',(1.,-5.00596043934455E-16,-5.57179392097267E-15));
#38359=DIRECTION('center_axis',(5.00596043934461E-16,1.,1.12027918221652E-15));
#38360=DIRECTION('ref_axis',(1.,-5.00596043934455E-16,-5.57179392097267E-15));
#38361=DIRECTION('center_axis',(5.00596043934461E-16,1.,1.12027918221652E-15));
#38362=DIRECTION('ref_axis',(0.828473350317593,2.12657775322542E-16,-0.560028488394602));
#38363=DIRECTION('',(0.779319883703892,1.08347942622894E-9,-0.626626299211701));
#38364=DIRECTION('',(5.57179392097267E-15,-1.12027918221652E-15,1.));
#38365=DIRECTION('center_axis',(-5.00596043934461E-16,-1.,-1.12027918221652E-15));
#38366=DIRECTION('ref_axis',(-5.57179392097267E-15,1.12027918221652E-15,
-1.));
#38367=DIRECTION('',(1.,-5.00596043934455E-16,-5.57179392097267E-15));
#38368=DIRECTION('',(-0.626626299195176,-2.0704530707019E-10,0.77931988371718));
#38369=DIRECTION('center_axis',(5.00596043934461E-16,1.,1.12027918221652E-15));
#38370=DIRECTION('ref_axis',(1.,-5.00596043934455E-16,-5.57179392097267E-15));
#38371=DIRECTION('center_axis',(5.00596043934461E-16,1.,1.12027918221652E-15));
#38372=DIRECTION('ref_axis',(1.,-5.00596043934455E-16,-5.57179392097267E-15));
#38373=DIRECTION('center_axis',(5.00596043934461E-16,1.,1.12027918221652E-15));
#38374=DIRECTION('ref_axis',(-0.560028488394602,1.20846949316291E-15,-0.828473350317593));
#38375=DIRECTION('',(-0.626626299212589,1.16622995081446E-9,-0.779319883703178));
#38376=DIRECTION('',(-5.57179392097267E-15,1.12027918221652E-15,-1.));
#38377=DIRECTION('',(0.779319883703586,-1.08364601666983E-9,0.626626299212081));
#38378=DIRECTION('center_axis',(5.00596043934461E-16,1.,1.12027918221652E-15));
#38379=DIRECTION('ref_axis',(1.,-5.00596043934455E-16,-5.57179392097267E-15));
#38380=DIRECTION('center_axis',(5.00596043934461E-16,1.,1.12027918221652E-15));
#38381=DIRECTION('ref_axis',(1.,-5.00596043934455E-16,-5.57179392097267E-15));
#38382=DIRECTION('center_axis',(5.00596043934461E-16,1.,1.12027918221652E-15));
#38383=DIRECTION('ref_axis',(-0.828473350317593,-2.12657775322542E-16,0.560028488394602));
#38384=DIRECTION('',(-0.779319883703892,1.08347879401104E-9,0.626626299211701));
#38385=DIRECTION('',(-5.57179392097267E-15,1.12027918221652E-15,-1.));
#38386=DIRECTION('center_axis',(-5.00596043934461E-16,-1.,-1.12027918221652E-15));
#38387=DIRECTION('ref_axis',(5.57179392097267E-15,-1.12027918221652E-15,
1.));
#38388=DIRECTION('',(-1.,5.00596043934455E-16,5.57179392097267E-15));
#38389=DIRECTION('',(0.626626299195176,-2.07044188331798E-10,-0.77931988371718));
#38390=DIRECTION('center_axis',(5.00596043934461E-16,1.,1.12027918221652E-15));
#38391=DIRECTION('ref_axis',(1.,-5.00596043934455E-16,-5.57179392097267E-15));
#38392=DIRECTION('center_axis',(5.00596043934461E-16,1.,1.12027918221652E-15));
#38393=DIRECTION('ref_axis',(1.,-5.00596043934455E-16,-5.57179392097267E-15));
#38394=DIRECTION('',(5.00596043934461E-16,1.,1.12027918221652E-15));
#38395=DIRECTION('center_axis',(5.00596043934461E-16,1.,1.12027918221652E-15));
#38396=DIRECTION('ref_axis',(1.,-5.00596043934455E-16,-5.57179392097267E-15));
#38397=DIRECTION('',(5.00596043934461E-16,1.,1.12027918221652E-15));
#38398=DIRECTION('center_axis',(5.00596043934461E-16,1.,1.12027918221652E-15));
#38399=DIRECTION('ref_axis',(1.,-5.00596043934455E-16,-5.57179392097267E-15));
#38400=DIRECTION('',(5.00596043934461E-16,1.,1.12027918221652E-15));
#38401=DIRECTION('center_axis',(5.00596043934461E-16,1.,1.12027918221652E-15));
#38402=DIRECTION('ref_axis',(1.,-5.00596043934455E-16,-5.57179392097267E-15));
#38403=DIRECTION('',(5.00596043934461E-16,1.,1.12027918221652E-15));
#38404=DIRECTION('center_axis',(5.00596043934461E-16,1.,1.12027918221652E-15));
#38405=DIRECTION('ref_axis',(-0.00546733966186705,-1.08624916607697E-15,
0.999985053986819));
#38406=DIRECTION('center_axis',(0.560028451650215,-2.46470073675675E-8,
-0.828473375155932));
#38407=DIRECTION('ref_axis',(-6.58554294166816E-9,-1.,2.52982371904519E-8));
#38408=DIRECTION('center_axis',(5.00596043934461E-16,1.,1.12027918221652E-15));
#38409=DIRECTION('ref_axis',(0.560028488394602,-1.20846949316291E-15,0.828473350317593));
#38410=DIRECTION('center_axis',(0.828473350319084,2.12657775319325E-16,
-0.560028488392396));
#38411=DIRECTION('ref_axis',(-2.1601502742123E-11,-1.,-3.19563778939926E-11));
#38412=DIRECTION('center_axis',(0.442362010728513,0.862800087335627,-0.244728136424609));
#38413=DIRECTION('ref_axis',(0.67492455342951,-0.499967312100476,-0.542687326191612));
#38414=DIRECTION('center_axis',(5.00596043934461E-16,1.,1.12027918221652E-15));
#38415=DIRECTION('ref_axis',(-5.57179392097266E-15,1.12027918221652E-15,
-1.));
#38416=DIRECTION('center_axis',(5.00596043934461E-16,1.,1.12027918221652E-15));
#38417=DIRECTION('ref_axis',(5.57179392097266E-15,-1.12027918221652E-15,
1.));
#38418=DIRECTION('',(-5.00596043934461E-16,-1.,-1.12027918221652E-15));
#38419=DIRECTION('center_axis',(5.00596043934461E-16,1.,1.12027918221652E-15));
#38420=DIRECTION('ref_axis',(5.57179392097266E-15,-1.12027918221652E-15,
1.));
#38421=DIRECTION('center_axis',(5.00596043934461E-16,1.,1.12027918221652E-15));
#38422=DIRECTION('ref_axis',(0.875020006168853,-9.80343870285712E-16,0.484086757517968));
#38423=DIRECTION('center_axis',(5.00596043934461E-16,1.,1.12027918221652E-15));
#38424=DIRECTION('ref_axis',(0.828473350317593,2.12657775322542E-16,-0.560028488394602));
#38425=DIRECTION('center_axis',(5.00596043934461E-16,1.,1.12027918221652E-15));
#38426=DIRECTION('ref_axis',(-5.57179392097266E-15,1.12027918221652E-15,
-1.));
#38427=DIRECTION('center_axis',(5.00596043934461E-16,1.,1.12027918221652E-15));
#38428=DIRECTION('ref_axis',(-0.560028488394602,1.20846949316291E-15,-0.828473350317593));
#38429=DIRECTION('center_axis',(5.00596043934461E-16,1.,1.12027918221652E-15));
#38430=DIRECTION('ref_axis',(-0.875020006168853,9.80343870285712E-16,-0.484086757517968));
#38431=DIRECTION('center_axis',(5.00596043934461E-16,1.,1.12027918221652E-15));
#38432=DIRECTION('ref_axis',(-0.828473350317593,-2.12657775322542E-16,0.560028488394602));
#38433=DIRECTION('center_axis',(5.00596043934461E-16,1.,1.12027918221652E-15));
#38434=DIRECTION('ref_axis',(5.57179392097266E-15,-1.12027918221652E-15,
1.));
#38435=DIRECTION('center_axis',(5.00596043934461E-16,1.,1.12027918221652E-15));
#38436=DIRECTION('ref_axis',(5.57179392097266E-15,-1.12027918221652E-15,
1.));
#38437=DIRECTION('center_axis',(5.00596043934461E-16,1.,1.12027918221652E-15));
#38438=DIRECTION('ref_axis',(-0.00546733966186705,-1.08624916607697E-15,
0.999985053986819));
#38439=DIRECTION('center_axis',(-5.00596043934461E-16,-1.,-1.12027918221652E-15));
#38440=DIRECTION('ref_axis',(0.484075514152618,-1.22259995249413E-15,0.875026226234322));
#38441=DIRECTION('center_axis',(0.875024443058473,1.04269557576734E-16,
-0.484078737448991));
#38442=DIRECTION('ref_axis',(-5.00596043934461E-16,-1.,-1.12027918221652E-15));
#38443=DIRECTION('center_axis',(0.875024443058478,-9.80337106658779E-16,
0.484078737448981));
#38444=DIRECTION('ref_axis',(-5.00596043934461E-16,-1.,-1.12027918221652E-15));
#38445=DIRECTION('center_axis',(5.00596043934461E-16,1.,1.12027918221652E-15));
#38446=DIRECTION('ref_axis',(1.,-5.00596043934455E-16,-5.57179392097267E-15));
#38447=DIRECTION('',(0.626626299213187,8.21459917499281E-8,-0.779319883702693));
#38448=DIRECTION('',(-1.,-7.69979604021266E-13,5.5717939209718E-15));
#38449=DIRECTION('',(0.626626299213087,-8.21413452539801E-8,0.779319883702774));
#38450=DIRECTION('center_axis',(5.00596043934461E-16,1.,1.12027918221652E-15));
#38451=DIRECTION('ref_axis',(1.,-5.00596043934455E-16,-5.57179392097267E-15));
#38452=DIRECTION('center_axis',(5.00596043934461E-16,1.,1.12027918221652E-15));
#38453=DIRECTION('ref_axis',(0.875024725126116,-9.80336676666241E-16,0.484078227581002));
#38454=DIRECTION('',(-0.779319883702693,8.21478081333498E-8,-0.626626299213187));
#38455=DIRECTION('',(5.57179392097228E-15,-7.71593186762516E-13,1.));
#38456=DIRECTION('',(0.779319883702774,-8.21427723649357E-8,-0.626626299213086));
#38457=DIRECTION('center_axis',(5.00596043934461E-16,1.,1.12027918221652E-15));
#38458=DIRECTION('ref_axis',(1.,-5.00596043934455E-16,-5.57179392097267E-15));
#38459=DIRECTION('center_axis',(-5.00596043934461E-16,-1.,-1.12027918221652E-15));
#38460=DIRECTION('ref_axis',(-0.484075514152618,1.22259995249413E-15,-0.875026226234322));
#38461=DIRECTION('',(-0.626626299213187,8.21459906311898E-8,0.779319883702693));
#38462=DIRECTION('',(1.,-7.70973503624234E-13,-5.57179392097353E-15));
#38463=DIRECTION('',(-0.626626299213087,-8.21413428804951E-8,-0.779319883702774));
#38464=DIRECTION('center_axis',(5.00596043934461E-16,1.,1.12027918221652E-15));
#38465=DIRECTION('ref_axis',(1.,-5.00596043934455E-16,-5.57179392097267E-15));
#38466=DIRECTION('center_axis',(5.00596043934461E-16,1.,1.12027918221652E-15));
#38467=DIRECTION('ref_axis',(-0.875025039198583,9.80336197883637E-16,-0.484077659859984));
#38468=DIRECTION('',(0.779319883702693,8.21474230077581E-8,0.626626299213187));
#38469=DIRECTION('',(-5.57179392097305E-15,-7.69352628398084E-13,-1.));
#38470=DIRECTION('',(-0.779319883702773,-8.21432340431895E-8,0.626626299213087));
#38471=DIRECTION('center_axis',(0.626626299211202,-1.18674248841174E-15,
0.779319883704293));
#38472=DIRECTION('ref_axis',(-5.00596043934461E-16,-1.,-1.12027918221652E-15));
#38473=DIRECTION('center_axis',(-0.626626299211202,1.18674248841174E-15,
-0.779319883704293));
#38474=DIRECTION('ref_axis',(0.674910816962253,-0.499999999999999,-0.542674293796331));
#38475=DIRECTION('',(0.626626006620295,2.71817970602453E-7,0.779320118967185));
#38476=DIRECTION('center_axis',(0.887935155463387,-0.383064347768995,0.254622986316092));
#38477=DIRECTION('ref_axis',(0.125932648739722,-0.329956706076109,-0.935558410841783));
#38478=DIRECTION('center_axis',(0.626626299211202,-1.18674248841174E-15,
0.779319883704293));
#38479=DIRECTION('ref_axis',(5.00596043934461E-16,1.,1.12027918221652E-15));
#38480=DIRECTION('center_axis',(-0.626626299211202,1.18674248841174E-15,
-0.779319883704293));
#38481=DIRECTION('ref_axis',(-0.674910816962253,0.499999999999999,0.542674293796331));
#38482=DIRECTION('center_axis',(-0.705697508381116,0.522807970064417,-0.478187048237203));
#38483=DIRECTION('ref_axis',(-0.384232653056518,0.284654389439118,0.87825801840814));
#38484=DIRECTION('center_axis',(-0.595274941165209,-0.803522087077111,2.41658023188801E-15));
#38485=DIRECTION('ref_axis',(5.39575063434723E-7,-3.99734514942978E-7,0.999999999999775));
#38486=DIRECTION('center_axis',(-1.,5.00596043934455E-16,5.57179392097267E-15));
#38487=DIRECTION('ref_axis',(5.57179392097266E-15,-1.12027918221652E-15,
1.));
#38488=DIRECTION('center_axis',(-1.,5.00596043934455E-16,5.57179392097267E-15));
#38489=DIRECTION('ref_axis',(5.57179392097266E-15,-1.12027918221652E-15,
1.));
#38490=DIRECTION('',(-0.999999999999992,-1.07234893281703E-7,-7.46977803037956E-8));
#38491=DIRECTION('center_axis',(-1.,5.00596043934455E-16,5.57179392097267E-15));
#38492=DIRECTION('ref_axis',(5.57179392097266E-15,-1.12027918221652E-15,
1.));
#38493=DIRECTION('center_axis',(5.00596043934461E-16,1.,1.12027918221652E-15));
#38494=DIRECTION('ref_axis',(0.999766740157022,0.,-0.0215978071989372));
#38495=DIRECTION('center_axis',(-5.00596043934461E-16,-1.,-1.12027918221652E-15));
#38496=DIRECTION('ref_axis',(1.,-5.00596043934455E-16,-5.57179392097267E-15));
#38497=DIRECTION('center_axis',(-2.79269672678808E-9,-1.12027918081851E-15,
1.));
#38498=DIRECTION('ref_axis',(1.,-5.00596047063061E-16,2.79269672678808E-9));
#38499=DIRECTION('center_axis',(5.00596043934461E-16,1.,1.12027918221652E-15));
#38500=DIRECTION('ref_axis',(1.,-5.00596043934455E-16,-5.57179392097267E-15));
#38501=DIRECTION('',(-5.14805905457061E-11,1.,1.12027918250336E-15));
#38502=DIRECTION('',(5.00596043688721E-16,1.,-4.41032069773478E-11));
#38503=DIRECTION('center_axis',(1.,-5.00596043934455E-16,-5.57179392097267E-15));
#38504=DIRECTION('ref_axis',(-5.57179392097267E-15,1.12027918221652E-15,
-1.));
#38505=DIRECTION('',(-7.46977803037955E-8,-1.07234894902578E-7,0.999999999999991));
#38506=DIRECTION('',(2.15527966388097E-12,-1.1202791822176E-15,1.));
#38507=DIRECTION('',(7.46713262143734E-8,1.0748494691062E-7,0.999999999999991));
#38508=DIRECTION('',(5.00596044221303E-16,1.,5.14822114209322E-11));
#38509=DIRECTION('center_axis',(5.57179392097266E-15,-1.12027918221652E-15,
1.));
#38510=DIRECTION('ref_axis',(1.,-5.00596043934455E-16,-5.57179392097267E-15));
#38511=DIRECTION('center_axis',(5.57179392097266E-15,-1.12027918221652E-15,
1.));
#38512=DIRECTION('ref_axis',(1.,-5.00596043934455E-16,-5.57179392097267E-15));
#38513=DIRECTION('center_axis',(5.57179392097266E-15,-1.12027918221652E-15,
1.));
#38514=DIRECTION('ref_axis',(1.,-5.00596043934455E-16,-5.57179392097267E-15));
#38515=DIRECTION('center_axis',(5.00596043934461E-16,1.,1.12027918221652E-15));
#38516=DIRECTION('ref_axis',(-0.0215978071989372,1.23572649697409E-15,-0.999766740157022));
#38517=DIRECTION('center_axis',(-5.00596043934461E-16,-1.,-1.12027918221652E-15));
#38518=DIRECTION('ref_axis',(-5.57179392097266E-15,1.12027918221652E-15,
-1.));
#38519=DIRECTION('center_axis',(1.,-5.0059604706306E-16,2.79269541533708E-9));
#38520=DIRECTION('ref_axis',(2.79269541533708E-9,1.12027918081851E-15,-1.));
#38521=DIRECTION('center_axis',(5.00596043934461E-16,1.,1.12027918221652E-15));
#38522=DIRECTION('ref_axis',(1.,-5.00596043934455E-16,-5.57179392097267E-15));
#38523=DIRECTION('',(-4.41048824446361E-11,1.,1.12027918246227E-15));
#38524=DIRECTION('center_axis',(-5.57179392097266E-15,1.12027918221652E-15,
-1.));
#38525=DIRECTION('ref_axis',(-1.,5.00596043934455E-16,5.57179392097267E-15));
#38526=DIRECTION('',(0.999999999999991,1.07484947530303E-7,-7.46713284325632E-8));
#38527=DIRECTION('',(1.,-5.00596043932047E-16,-2.15527966388097E-12));
#38528=DIRECTION('center_axis',(0.999999999999976,2.17635944148899E-7,-5.57179367715952E-15));
#38529=DIRECTION('ref_axis',(-5.75848107867473E-13,2.62032228371319E-6,
-0.999999999996567));
#38530=DIRECTION('center_axis',(-0.626626299211194,-5.59369195590911E-16,
0.7793198837043));
#38531=DIRECTION('ref_axis',(-5.00596043934461E-16,-1.,-1.12027918221652E-15));
#38532=DIRECTION('center_axis',(-0.626626299211194,-5.59369195590911E-16,
0.7793198837043));
#38533=DIRECTION('ref_axis',(-5.00596043934461E-16,-1.,-1.12027918221652E-15));
#38534=DIRECTION('',(-0.626626006343689,-2.71886424419567E-7,0.779320119189595));
#38535=DIRECTION('center_axis',(0.342295357878412,-0.707106781186532,-0.618735717390642));
#38536=DIRECTION('ref_axis',(-0.342295357878411,-0.707106781186553,0.618735717390618));
#38537=DIRECTION('center_axis',(-0.875024443058478,9.80337106658779E-16,
-0.484078737448981));
#38538=DIRECTION('ref_axis',(-5.00596043934461E-16,-1.,-1.12027918221652E-15));
#38539=DIRECTION('center_axis',(-0.442362657739701,-0.862799639016597,-0.244728547477197));
#38540=DIRECTION('ref_axis',(0.674924135928914,-0.49996807137079,0.542687145923303));
#38541=DIRECTION('center_axis',(-0.82847335444329,2.83557470020383E-8,-0.560028482291286));
#38542=DIRECTION('ref_axis',(-2.28233127966104E-8,-1.,-1.68692143143682E-8));
#38543=DIRECTION('center_axis',(-0.626626299211194,-5.59369195590911E-16,
0.7793198837043));
#38544=DIRECTION('ref_axis',(5.00596043934461E-16,1.,1.12027918221652E-15));
#38545=DIRECTION('center_axis',(-0.626626299211194,-5.59369195590911E-16,
0.7793198837043));
#38546=DIRECTION('ref_axis',(5.00596043934461E-16,1.,1.12027918221652E-15));
#38547=DIRECTION('center_axis',(0.,0.707106781186545,0.70710678118655));
#38548=DIRECTION('ref_axis',(0.,0.707106781186548,-0.707106781186548));
#38549=DIRECTION('center_axis',(1.,-5.00596043934455E-16,-5.57179392097267E-15));
#38550=DIRECTION('ref_axis',(-5.57179392097266E-15,1.12027918221652E-15,
-1.));
#38551=DIRECTION('center_axis',(1.,-5.00596043934455E-16,-5.57179392097267E-15));
#38552=DIRECTION('ref_axis',(-5.57179392097266E-15,1.12027918221652E-15,
-1.));
#38553=DIRECTION('center_axis',(5.00596043934461E-16,1.,1.12027918221652E-15));
#38554=DIRECTION('ref_axis',(-0.00546733966186705,-1.08624916607697E-15,
0.999985053986819));
#38555=DIRECTION('center_axis',(-0.560028488398899,1.2084694931618E-15,
-0.828473350314689));
#38556=DIRECTION('ref_axis',(-7.44149101541802E-12,-1.,5.02881413593191E-12));
#38557=DIRECTION('center_axis',(-0.244728038654104,0.862800306783108,-0.442361636799001));
#38558=DIRECTION('ref_axis',(-0.542687484719605,-0.499966948603119,-0.674924695231397));
#38559=DIRECTION('center_axis',(0.779319883704293,3.11871947293856E-16,
-0.626626299211202));
#38560=DIRECTION('ref_axis',(5.00596043934461E-16,1.,1.12027918221652E-15));
#38561=DIRECTION('',(0.779320120962128,2.74269932471282E-7,-0.62662600413923));
#38562=DIRECTION('center_axis',(-0.779319883704293,-3.11871947293856E-16,
0.626626299211202));
#38563=DIRECTION('ref_axis',(0.54267429379633,0.499999999999998,0.674910816962253));
#38564=DIRECTION('center_axis',(-0.478187048237203,0.522807970064417,0.705697508381116));
#38565=DIRECTION('ref_axis',(0.87825801840814,0.284654389439118,0.384232653056518));
#38566=DIRECTION('center_axis',(2.91450932048691E-15,-0.803522087077112,
0.595274941165208));
#38567=DIRECTION('ref_axis',(0.999999999999775,-3.99734512055927E-7,-5.39575060374155E-7));
#38568=DIRECTION('center_axis',(5.57179392097266E-15,-1.12027918221652E-15,
1.));
#38569=DIRECTION('ref_axis',(1.,-5.00596043934455E-16,-5.57179392097267E-15));
#38570=DIRECTION('center_axis',(5.57179392097266E-15,-1.12027918221652E-15,
1.));
#38571=DIRECTION('ref_axis',(1.,-5.00596043934455E-16,-5.57179392097267E-15));
#38572=DIRECTION('center_axis',(5.57179402992023E-15,2.17635943782516E-7,
0.999999999999976));
#38573=DIRECTION('ref_axis',(0.999999999996567,2.62032228244231E-6,-5.75848106983604E-13));
#38574=DIRECTION('center_axis',(-0.7793198837043,1.09212084877752E-15,-0.626626299211194));
#38575=DIRECTION('ref_axis',(-5.00596043934461E-16,-1.,-1.12027918221652E-15));
#38576=DIRECTION('center_axis',(-0.7793198837043,1.09212084877752E-15,-0.626626299211194));
#38577=DIRECTION('ref_axis',(-5.00596043934461E-16,-1.,-1.12027918221652E-15));
#38578=DIRECTION('',(-0.779320120541394,-2.73779246727676E-7,-0.626626004662488));
#38579=DIRECTION('center_axis',(0.618735717390639,-0.707106781186534,0.342295357878411));
#38580=DIRECTION('ref_axis',(-0.618735717390618,-0.707106781186553,-0.342295357878411));
#38581=DIRECTION('center_axis',(0.484078737448981,7.3794376656927E-16,-0.875024443058478));
#38582=DIRECTION('ref_axis',(-5.00596043934461E-16,-1.,-1.12027918221652E-15));
#38583=DIRECTION('center_axis',(0.244728012110787,-0.862800336285763,-0.442361593940383));
#38584=DIRECTION('ref_axis',(-0.542687494645365,-0.499966898890162,0.674924724076465));
#38585=DIRECTION('center_axis',(-0.7793198837043,1.09212084877752E-15,-0.626626299211194));
#38586=DIRECTION('ref_axis',(5.00596043934461E-16,1.,1.12027918221652E-15));
#38587=DIRECTION('center_axis',(-0.7793198837043,1.09212084877752E-15,-0.626626299211194));
#38588=DIRECTION('ref_axis',(5.00596043934461E-16,1.,1.12027918221652E-15));
#38589=DIRECTION('center_axis',(-0.70710678118655,0.707106781186545,0.));
#38590=DIRECTION('ref_axis',(0.70710678118655,0.707106781186545,0.));
#38591=DIRECTION('center_axis',(5.57179392097266E-15,-1.12027918221652E-15,
1.));
#38592=DIRECTION('ref_axis',(1.,-5.00596043934455E-16,-5.57179392097267E-15));
#38593=DIRECTION('center_axis',(5.57179392097266E-15,-1.12027918221652E-15,
1.));
#38594=DIRECTION('ref_axis',(1.,-5.00596043934455E-16,-5.57179392097267E-15));
#38595=DIRECTION('center_axis',(5.00596043934461E-16,1.,1.12027918221652E-15));
#38596=DIRECTION('ref_axis',(-0.00546733966186705,-1.08624916607697E-15,
0.999985053986819));
#38597=DIRECTION('center_axis',(-0.484078737448991,1.22259956840877E-15,
-0.875024443058473));
#38598=DIRECTION('ref_axis',(-5.00596043934461E-16,-1.,-1.12027918221652E-15));
#38599=DIRECTION('center_axis',(0.254622986316092,-0.383064347768995,-0.887935155463387));
#38600=DIRECTION('ref_axis',(-0.935558410841783,-0.329956706076109,-0.125932648739722));
#38601=DIRECTION('center_axis',(-0.779319883704293,-3.11871947293856E-16,
0.626626299211202));
#38602=DIRECTION('ref_axis',(-0.54267429379633,-0.499999999999998,-0.674910816962253));
#38603=DIRECTION('center_axis',(0.779319883704293,3.11871947293856E-16,
-0.626626299211202));
#38604=DIRECTION('ref_axis',(-5.00596043934461E-16,-1.,-1.12027918221652E-15));
#38605=DIRECTION('center_axis',(5.00596043934461E-16,1.,1.12027918221652E-15));
#38606=DIRECTION('ref_axis',(0.00546733966186705,1.08624916607697E-15,-0.999985053986819));
#38607=DIRECTION('center_axis',(-0.875024443058473,-1.04269557576734E-16,
0.484078737448991));
#38608=DIRECTION('ref_axis',(-5.00596043934461E-16,-1.,-1.12027918221652E-15));
#38609=DIRECTION('center_axis',(0.4423626577397,-0.862799639016598,0.244728547477196));
#38610=DIRECTION('ref_axis',(-0.674924135928915,-0.499968071370788,-0.542687145923305));
#38611=DIRECTION('center_axis',(0.82847335444329,2.83557475385409E-8,0.560028482291286));
#38612=DIRECTION('ref_axis',(2.28233165805793E-8,-1.,1.68692096745776E-8));
#38613=DIRECTION('center_axis',(0.626626299211194,5.59369195590911E-16,
-0.7793198837043));
#38614=DIRECTION('ref_axis',(5.00596043934461E-16,1.,1.12027918221652E-15));
#38615=DIRECTION('center_axis',(0.626626299211194,5.59369195590911E-16,
-0.7793198837043));
#38616=DIRECTION('ref_axis',(5.00596043934461E-16,1.,1.12027918221652E-15));
#38617=DIRECTION('',(0.626626006343689,-2.71886423154627E-7,-0.779320119189595));
#38618=DIRECTION('center_axis',(0.626626299211194,5.59369195590911E-16,
-0.7793198837043));
#38619=DIRECTION('ref_axis',(-5.00596043934461E-16,-1.,-1.12027918221652E-15));
#38620=DIRECTION('center_axis',(0.626626299211194,5.59369195590911E-16,
-0.7793198837043));
#38621=DIRECTION('ref_axis',(-5.00596043934461E-16,-1.,-1.12027918221652E-15));
#38622=DIRECTION('center_axis',(-0.342295357878412,-0.707106781186532,0.618735717390642));
#38623=DIRECTION('ref_axis',(0.342295357878402,-0.707106781186555,-0.618735717390621));
#38624=DIRECTION('center_axis',(-0.999999999999976,2.17635947033991E-7,
5.57179416478555E-15));
#38625=DIRECTION('ref_axis',(5.75848115427344E-13,2.62032228147263E-6,0.999999999996567));
#38626=DIRECTION('center_axis',(-1.,5.00596043934455E-16,5.57179392097267E-15));
#38627=DIRECTION('ref_axis',(5.57179392097266E-15,-1.12027918221652E-15,
1.));
#38628=DIRECTION('',(-1.,5.00596043932046E-16,2.15551302339697E-12));
#38629=DIRECTION('center_axis',(-1.,5.00596043934455E-16,5.57179392097267E-15));
#38630=DIRECTION('ref_axis',(5.57179392097266E-15,-1.12027918221652E-15,
1.));
#38631=DIRECTION('center_axis',(5.57179392097266E-15,-1.12027918221652E-15,
1.));
#38632=DIRECTION('ref_axis',(1.,-5.00596043934455E-16,-5.57179392097267E-15));
#38633=DIRECTION('',(-0.999999999999991,1.07484948739395E-7,7.46713262143735E-8));
#38634=DIRECTION('',(4.41048278525739E-11,1.,1.12027918197078E-15));
#38635=DIRECTION('center_axis',(5.00596043934461E-16,1.,1.12027918221652E-15));
#38636=DIRECTION('ref_axis',(-0.707106781189596,-4.38182149261264E-16,0.707106781183499));
#38637=DIRECTION('center_axis',(-5.00596043934461E-16,-1.,-1.12027918221652E-15));
#38638=DIRECTION('ref_axis',(5.57179392097266E-15,-1.12027918221652E-15,
1.));
#38639=DIRECTION('',(5.00596043647619E-16,1.,-5.14799708625678E-11));
#38640=DIRECTION('center_axis',(5.00596043934461E-16,1.,1.12027918221652E-15));
#38641=DIRECTION('ref_axis',(0.0215978071989347,-1.23572649697409E-15,0.999766740157022));
#38642=DIRECTION('center_axis',(-1.,5.00596047063061E-16,-2.79269621677908E-9));
#38643=DIRECTION('ref_axis',(-2.79269621677908E-9,-1.12027918081851E-15,
1.));
#38644=DIRECTION('center_axis',(-5.57179392097266E-15,1.12027918221652E-15,
-1.));
#38645=DIRECTION('ref_axis',(-1.,5.00596043934455E-16,5.57179392097267E-15));
#38646=DIRECTION('center_axis',(-5.57179392097266E-15,1.12027918221652E-15,
-1.));
#38647=DIRECTION('ref_axis',(-1.,5.00596043934455E-16,5.57179392097267E-15));
#38648=DIRECTION('center_axis',(-5.57179392097266E-15,1.12027918221652E-15,
-1.));
#38649=DIRECTION('ref_axis',(-1.,5.00596043934455E-16,5.57179392097267E-15));
#38650=DIRECTION('',(7.46977803037954E-8,-1.0723489266202E-7,-0.999999999999991));
#38651=DIRECTION('center_axis',(-1.,5.00596043934455E-16,5.57179392097267E-15));
#38652=DIRECTION('ref_axis',(5.57179392097267E-15,-1.12027918221652E-15,
1.));
#38653=DIRECTION('',(-2.15527966388097E-12,1.1202791822176E-15,-1.));
#38654=DIRECTION('',(-7.46713339879133E-8,1.07302226011078E-7,-0.999999999999991));
#38655=DIRECTION('center_axis',(-5.57179392097266E-15,1.12027918221652E-15,
-1.));
#38656=DIRECTION('ref_axis',(-1.,5.00596043934455E-16,5.57179392097267E-15));
#38657=DIRECTION('center_axis',(-5.57179392097266E-15,1.12027918221652E-15,
-1.));
#38658=DIRECTION('ref_axis',(-1.,5.00596043934455E-16,5.57179392097267E-15));
#38659=DIRECTION('center_axis',(-0.47818704823722,-0.522807970064411,-0.705697508381108));
#38660=DIRECTION('ref_axis',(-0.87825801840813,0.284654389439118,0.38423265305654));
#38661=DIRECTION('center_axis',(0.7793198837043,-1.09212084877752E-15,0.626626299211194));
#38662=DIRECTION('ref_axis',(5.00596043934461E-16,1.,1.12027918221652E-15));
#38663=DIRECTION('center_axis',(-2.91450932149465E-15,0.803522086951483,
-0.595274941334786));
#38664=DIRECTION('ref_axis',(-0.999999999999775,-3.99555386113565E-7,-5.39333260137364E-7));
#38665=DIRECTION('center_axis',(0.7793198837043,-1.09212084877752E-15,0.626626299211194));
#38666=DIRECTION('ref_axis',(5.00596043934461E-16,1.,1.12027918221652E-15));
#38667=DIRECTION('',(0.779320120539837,-2.73783421093733E-7,0.626626004664424));
#38668=DIRECTION('center_axis',(-0.244728012110788,-0.862800336285764,0.442361593940382));
#38669=DIRECTION('ref_axis',(0.542687494645364,-0.499966898890161,-0.674924724076466));
#38670=DIRECTION('center_axis',(-0.560028451650283,-2.46469991572629E-8,
0.828473375155886));
#38671=DIRECTION('ref_axis',(6.58553923956407E-9,-1.,-2.52982297828268E-8));
#38672=DIRECTION('center_axis',(5.00596043934461E-16,1.,1.12027918221652E-15));
#38673=DIRECTION('ref_axis',(0.00546733966186705,1.08624916607697E-15,-0.999985053986819));
#38674=DIRECTION('center_axis',(-0.828473350319084,-2.12657775319325E-16,
0.560028488392396));
#38675=DIRECTION('ref_axis',(2.16005015500351E-11,-1.,3.19541373356282E-11));
#38676=DIRECTION('center_axis',(-0.442362010728512,0.862800087335627,0.244728136424611));
#38677=DIRECTION('ref_axis',(-0.674924553429511,-0.499967312100476,0.542687326191611));
#38678=DIRECTION('center_axis',(-0.626626299211202,1.18674248841174E-15,
-0.779319883704293));
#38679=DIRECTION('ref_axis',(5.00596043934461E-16,1.,1.12027918221652E-15));
#38680=DIRECTION('',(-0.626626006620295,2.71817973008439E-7,-0.779320118967185));
#38681=DIRECTION('center_axis',(0.626626299211202,-1.18674248841174E-15,
0.779319883704293));
#38682=DIRECTION('ref_axis',(0.674910816962253,0.499999999999999,-0.54267429379633));
#38683=DIRECTION('center_axis',(0.705697508381122,0.522807970064412,0.478187048237199));
#38684=DIRECTION('ref_axis',(0.384232653056518,0.284654389439118,-0.87825801840814));
#38685=DIRECTION('center_axis',(0.595274941165208,-0.803522087077112,-4.21691836509533E-15));
#38686=DIRECTION('ref_axis',(-5.39575061594927E-7,-3.99734511339439E-7,
-0.999999999999775));
#38687=DIRECTION('center_axis',(1.,-5.00596043934455E-16,-5.57179392097267E-15));
#38688=DIRECTION('ref_axis',(-5.57179392097266E-15,1.12027918221652E-15,
-1.));
#38689=DIRECTION('center_axis',(1.,-5.00596043934455E-16,-5.57179392097267E-15));
#38690=DIRECTION('ref_axis',(-5.57179392097266E-15,1.12027918221652E-15,
-1.));
#38691=DIRECTION('center_axis',(-0.626626299211202,1.18674248841174E-15,
-0.779319883704293));
#38692=DIRECTION('ref_axis',(-5.00596043934461E-16,-1.,-1.12027918221652E-15));
#38693=DIRECTION('center_axis',(0.626626299211202,-1.18674248841174E-15,
0.779319883704293));
#38694=DIRECTION('ref_axis',(-0.674910816962253,-0.499999999999999,0.54267429379633));
#38695=DIRECTION('center_axis',(-0.887935155463387,-0.383064347768995,-0.254622986316092));
#38696=DIRECTION('ref_axis',(-0.125932648739722,-0.329956706076109,0.935558410841783));
#38697=DIRECTION('center_axis',(-0.618735717390635,-0.707106781186537,-0.342295357878415));
#38698=DIRECTION('ref_axis',(0.618735717390611,-0.707106781186558,0.342295357878414));
#38699=DIRECTION('center_axis',(0.7793198837043,-1.09212084877752E-15,0.626626299211194));
#38700=DIRECTION('ref_axis',(-5.00596043934461E-16,-1.,-1.12027918221652E-15));
#38701=DIRECTION('center_axis',(-0.484078737448981,-7.3794376656927E-16,
0.875024443058478));
#38702=DIRECTION('ref_axis',(-5.00596043934461E-16,-1.,-1.12027918221652E-15));
#38703=DIRECTION('center_axis',(0.7793198837043,-1.09212084877752E-15,0.626626299211194));
#38704=DIRECTION('ref_axis',(-5.00596043934461E-16,-1.,-1.12027918221652E-15));
#38705=DIRECTION('center_axis',(-5.57179381202484E-15,2.17635945960674E-7,
-0.999999999999976));
#38706=DIRECTION('ref_axis',(-0.999999999996567,2.62032228309351E-6,5.75848112614908E-13));
#38707=DIRECTION('center_axis',(-5.57179392097266E-15,1.12027918221652E-15,
-1.));
#38708=DIRECTION('ref_axis',(-1.,5.00596043934455E-16,5.57179392097267E-15));
#38709=DIRECTION('center_axis',(-5.57179392097266E-15,1.12027918221652E-15,
-1.));
#38710=DIRECTION('ref_axis',(-1.,5.00596043934455E-16,5.57179392097267E-15));
#38711=DIRECTION('center_axis',(-3.71898927649643E-15,-0.803522087077111,
-0.59527494116521));
#38712=DIRECTION('ref_axis',(-0.999999999999775,-3.9973451068302E-7,5.395750598724E-7));
#38713=DIRECTION('center_axis',(-0.779319883704293,-3.11871947293856E-16,
0.626626299211202));
#38714=DIRECTION('ref_axis',(-5.00596043934461E-16,-1.,-1.12027918221652E-15));
#38715=DIRECTION('center_axis',(0.779319883704293,3.11871947293856E-16,
-0.626626299211202));
#38716=DIRECTION('ref_axis',(0.54267429379633,-0.5,0.674910816962252));
#38717=DIRECTION('',(-0.779320120961903,2.7427056598253E-7,0.62662600413951));
#38718=DIRECTION('center_axis',(0.618735717390635,0.707106781186537,-0.342295357878415));
#38719=DIRECTION('ref_axis',(0.618735717390611,-0.707106781186558,-0.342295357878414));
#38720=DIRECTION('center_axis',(0.24472801409699,0.862800334966154,0.442361595415376));
#38721=DIRECTION('ref_axis',(0.542687498153732,-0.499966900858982,0.674924719797037));
#38722=DIRECTION('center_axis',(0.484078737448991,-1.22259956840877E-15,
0.875024443058473));
#38723=DIRECTION('ref_axis',(-5.00596043934461E-16,-1.,-1.12027918221652E-15));
#38724=DIRECTION('center_axis',(5.00596043934461E-16,1.,1.12027918221652E-15));
#38725=DIRECTION('ref_axis',(0.00546733966186705,1.08624916607697E-15,-0.999985053986819));
#38726=DIRECTION('center_axis',(0.560028488398899,-1.2084694931618E-15,
0.828473350314689));
#38727=DIRECTION('ref_axis',(7.44048982333015E-12,-1.,-5.03105469429634E-12));
#38728=DIRECTION('center_axis',(5.00596043934461E-16,1.,1.12027918221652E-15));
#38729=DIRECTION('ref_axis',(0.00546733966186705,1.08624916607697E-15,-0.999985053986819));
#38730=DIRECTION('center_axis',(-0.779319883704293,-3.11871947293856E-16,
0.626626299211202));
#38731=DIRECTION('ref_axis',(5.00596043934461E-16,1.,1.12027918221652E-15));
#38732=DIRECTION('center_axis',(0.779319883704293,3.11871947293856E-16,
-0.626626299211202));
#38733=DIRECTION('ref_axis',(-0.54267429379633,0.5,-0.674910816962252));
#38734=DIRECTION('center_axis',(0.478187048237211,0.522807970064414,-0.705697508381112));
#38735=DIRECTION('ref_axis',(-0.878258018408137,0.284654389439121,-0.384232653056521));
#38736=DIRECTION('center_axis',(-1.,5.00596043934455E-16,5.57179392097267E-15));
#38737=DIRECTION('ref_axis',(5.57179392097266E-15,-1.12027918221652E-15,
1.));
#38738=DIRECTION('center_axis',(-1.,5.00596043934455E-16,5.57179392097267E-15));
#38739=DIRECTION('ref_axis',(5.57179392097266E-15,-1.12027918221652E-15,
1.));
#38740=DIRECTION('center_axis',(0.,0.707106781186545,-0.70710678118655));
#38741=DIRECTION('ref_axis',(0.,0.707106781186545,0.70710678118655));
#38742=DIRECTION('center_axis',(5.00596043934461E-16,1.,1.12027918221652E-15));
#38743=DIRECTION('ref_axis',(0.00546733966186688,1.05265590482978E-15,-0.999985053986819));
#38744=DIRECTION('center_axis',(5.00596043934461E-16,1.,1.12027918221652E-15));
#38745=DIRECTION('ref_axis',(-5.57179392097267E-15,1.12027918221652E-15,
-1.));
#38746=DIRECTION('center_axis',(0.999985053986819,-5.06713508824686E-16,
0.00546733966186613));
#38747=DIRECTION('ref_axis',(-0.00546733966186613,-1.12784561231762E-15,
0.999985053986819));
#38748=DIRECTION('center_axis',(5.00596043934461E-16,1.,1.12027918221652E-15));
#38749=DIRECTION('ref_axis',(-5.57179392097267E-15,1.12027918221652E-15,
-1.));
#38750=DIRECTION('center_axis',(-5.00596043934461E-16,-1.,-1.12027918221652E-15));
#38751=DIRECTION('ref_axis',(-5.57179392097266E-15,1.12027918221652E-15,
-1.));
#38752=DIRECTION('center_axis',(5.00596043934461E-16,1.,1.12027918221652E-15));
#38753=DIRECTION('ref_axis',(-0.0102648972912855,1.04414803197664E-15,-0.999947314553922));
#38754=DIRECTION('center_axis',(5.00596043934461E-16,1.,1.12027918221652E-15));
#38755=DIRECTION('ref_axis',(5.57179392097266E-15,-1.12027918221652E-15,
1.));
#38756=DIRECTION('center_axis',(5.00596043934461E-16,1.,1.12027918221652E-15));
#38757=DIRECTION('ref_axis',(5.57179392097266E-15,-1.12027918221652E-15,
1.));
#38758=DIRECTION('center_axis',(0.999947314553922,-4.89070119065563E-16,
-0.0102648972912858));
#38759=DIRECTION('ref_axis',(0.0102648972912858,-1.08765419997566E-15,0.999947314553921));
#38760=DIRECTION('center_axis',(5.00596043934461E-16,1.,1.12027918221652E-15));
#38761=DIRECTION('ref_axis',(-5.57179392097266E-15,1.12027918221652E-15,
-1.));
#38762=DIRECTION('center_axis',(-5.00596043934461E-16,-1.,-1.12027918221652E-15));
#38763=DIRECTION('ref_axis',(5.57179392097266E-15,-1.12027918221652E-15,
1.));
#38764=DIRECTION('',(-5.00596043934461E-16,-1.,-1.12027918221652E-15));
#38765=DIRECTION('center_axis',(5.00596043934461E-16,1.,1.12027918221652E-15));
#38766=DIRECTION('ref_axis',(-5.57179392097267E-15,1.12027918221652E-15,
-1.));
#38767=DIRECTION('center_axis',(-5.00596043934461E-16,-1.,-1.12027918221652E-15));
#38768=DIRECTION('ref_axis',(5.57179392097266E-15,-1.12027918221652E-15,
1.));
#38769=DIRECTION('center_axis',(5.00596043934461E-16,1.,1.12027918221652E-15));
#38770=DIRECTION('ref_axis',(-5.57179392097266E-15,1.12027918221652E-15,
-1.));
#38771=DIRECTION('center_axis',(-5.00596043934461E-16,-1.,-1.12027918221652E-15));
#38772=DIRECTION('ref_axis',(5.57179392097266E-15,-1.12027918221652E-15,
1.));
#38773=DIRECTION('',(5.00596043934461E-16,1.,1.12027918221652E-15));
#38774=DIRECTION('center_axis',(5.00596043934461E-16,1.,1.12027918221652E-15));
#38775=DIRECTION('ref_axis',(-5.57179392097267E-15,1.12027918221652E-15,
-1.));
#38776=DIRECTION('center_axis',(-5.00596043934461E-16,-1.,-1.12027918221652E-15));
#38777=DIRECTION('ref_axis',(5.57179392097266E-15,-1.12027918221652E-15,
1.));
#38778=DIRECTION('center_axis',(5.00596043934461E-16,1.,1.12027918221652E-15));
#38779=DIRECTION('ref_axis',(-5.57179392097266E-15,1.12027918221652E-15,
-1.));
#38780=DIRECTION('center_axis',(-5.00596043934461E-16,-1.,-1.12027918221652E-15));
#38781=DIRECTION('ref_axis',(5.57179392097266E-15,-1.12027918221652E-15,
1.));
#38782=DIRECTION('',(-5.00596043934461E-16,-1.,-1.12027918221652E-15));
#38783=DIRECTION('center_axis',(5.00596043934461E-16,1.,1.12027918221652E-15));
#38784=DIRECTION('ref_axis',(-5.57179392097267E-15,1.12027918221652E-15,
-1.));
#38785=DIRECTION('center_axis',(-5.00596043934461E-16,-1.,-1.12027918221652E-15));
#38786=DIRECTION('ref_axis',(5.57179392097266E-15,-1.12027918221652E-15,
1.));
#38787=DIRECTION('center_axis',(5.00596043934461E-16,1.,1.12027918221652E-15));
#38788=DIRECTION('ref_axis',(-5.57179392097266E-15,1.12027918221652E-15,
-1.));
#38789=DIRECTION('center_axis',(-5.00596043934461E-16,-1.,-1.12027918221652E-15));
#38790=DIRECTION('ref_axis',(5.57179392097266E-15,-1.12027918221652E-15,
1.));
#38791=DIRECTION('',(5.00596043934461E-16,1.,1.12027918221652E-15));
#38792=DIRECTION('center_axis',(5.00596043934461E-16,1.,1.12027918221652E-15));
#38793=DIRECTION('ref_axis',(-5.57179392097267E-15,1.12027918221652E-15,
-1.));
#38794=DIRECTION('center_axis',(-5.00596043934461E-16,-1.,-1.12027918221652E-15));
#38795=DIRECTION('ref_axis',(5.57179392097266E-15,-1.12027918221652E-15,
1.));
#38796=DIRECTION('center_axis',(5.00596043934461E-16,1.,1.12027918221652E-15));
#38797=DIRECTION('ref_axis',(-5.57179392097266E-15,1.12027918221652E-15,
-1.));
#38798=DIRECTION('center_axis',(-5.00596043934461E-16,-1.,-1.12027918221652E-15));
#38799=DIRECTION('ref_axis',(5.57179392097266E-15,-1.12027918221652E-15,
1.));
#38800=DIRECTION('',(-5.00596043934461E-16,-1.,-1.12027918221652E-15));
#38801=DIRECTION('center_axis',(5.00596043934461E-16,1.,1.12027918221652E-15));
#38802=DIRECTION('ref_axis',(-5.57179392097267E-15,1.12027918221652E-15,
-1.));
#38803=DIRECTION('center_axis',(-5.00596043934461E-16,-1.,-1.12027918221652E-15));
#38804=DIRECTION('ref_axis',(5.57179392097266E-15,-1.12027918221652E-15,
1.));
#38805=DIRECTION('center_axis',(5.00596043934461E-16,1.,1.12027918221652E-15));
#38806=DIRECTION('ref_axis',(-5.57179392097266E-15,1.12027918221652E-15,
-1.));
#38807=DIRECTION('center_axis',(-5.00596043934461E-16,-1.,-1.12027918221652E-15));
#38808=DIRECTION('ref_axis',(5.57179392097266E-15,-1.12027918221652E-15,
1.));
#38809=DIRECTION('',(5.00596043934461E-16,1.,1.12027918221652E-15));
#38810=DIRECTION('center_axis',(5.00596043934461E-16,1.,1.12027918221652E-15));
#38811=DIRECTION('ref_axis',(-5.57179392097267E-15,1.12027918221652E-15,
-1.));
#38812=DIRECTION('center_axis',(-5.00596043934461E-16,-1.,-1.12027918221652E-15));
#38813=DIRECTION('ref_axis',(-1.,5.00596043934455E-16,5.57179392097267E-15));
#38814=DIRECTION('center_axis',(5.00596043934461E-16,1.,1.12027918221652E-15));
#38815=DIRECTION('ref_axis',(-5.57179392097266E-15,1.12027918221652E-15,
-1.));
#38816=DIRECTION('center_axis',(5.00596043934461E-16,1.,1.12027918221652E-15));
#38817=DIRECTION('ref_axis',(1.,-5.00596043934455E-16,-5.57179392097267E-15));
#38818=DIRECTION('',(5.00596043934461E-16,1.,1.12027918221652E-15));
#38819=DIRECTION('center_axis',(-5.00596043934461E-16,-1.,-1.12027918221652E-15));
#38820=DIRECTION('ref_axis',(-1.,5.00596043934455E-16,5.57179392097267E-15));
#38821=DIRECTION('center_axis',(5.00596043934461E-16,1.,1.12027918221652E-15));
#38822=DIRECTION('ref_axis',(-1.,5.00596043934455E-16,5.57179392097267E-15));
#38823=DIRECTION('',(5.57179392097266E-15,-1.12027918221652E-15,1.));
#38824=DIRECTION('center_axis',(5.00596043934461E-16,1.,1.12027918221652E-15));
#38825=DIRECTION('ref_axis',(-5.57179392097266E-15,1.12027918221652E-15,
-1.));
#38826=DIRECTION('',(-1.,5.00596043934455E-16,5.57179392097266E-15));
#38827=DIRECTION('center_axis',(5.00596043934461E-16,1.,1.12027918221652E-15));
#38828=DIRECTION('ref_axis',(1.,-5.00596043934455E-16,-5.57179392097267E-15));
#38829=DIRECTION('',(-5.57179392097266E-15,1.12027918221652E-15,-1.));
#38830=DIRECTION('center_axis',(5.00596043934461E-16,1.,1.12027918221652E-15));
#38831=DIRECTION('ref_axis',(5.57179392097266E-15,-1.12027918221652E-15,
1.));
#38832=DIRECTION('',(1.,-5.00596043934455E-16,-5.57179392097266E-15));
#38833=DIRECTION('center_axis',(-5.00596043934461E-16,-1.,-1.12027918221652E-15));
#38834=DIRECTION('ref_axis',(-1.,5.00596043934455E-16,5.57179392097267E-15));
#38835=DIRECTION('',(5.00596043934461E-16,1.,1.12027918221652E-15));
#38836=DIRECTION('',(5.00596043934461E-16,1.,1.12027918221652E-15));
#38837=DIRECTION('center_axis',(-5.57179392097266E-15,1.12027918221652E-15,
-1.));
#38838=DIRECTION('ref_axis',(1.,-5.00596043934455E-16,-5.57179392097267E-15));
#38839=DIRECTION('',(5.00596043934461E-16,1.,1.12027918221652E-15));
#38840=DIRECTION('center_axis',(-5.00596043934461E-16,-1.,-1.12027918221652E-15));
#38841=DIRECTION('ref_axis',(-1.,5.00596043934455E-16,5.57179392097267E-15));
#38842=DIRECTION('',(5.00596043934461E-16,1.,1.12027918221652E-15));
#38843=DIRECTION('center_axis',(-1.,5.00596043934455E-16,5.57179392097267E-15));
#38844=DIRECTION('ref_axis',(-5.57179392097267E-15,1.12027918221652E-15,
-1.));
#38845=DIRECTION('',(5.00596043934461E-16,1.,1.12027918221652E-15));
#38846=DIRECTION('center_axis',(-5.00596043934461E-16,-1.,-1.12027918221652E-15));
#38847=DIRECTION('ref_axis',(-1.,5.00596043934455E-16,5.57179392097267E-15));
#38848=DIRECTION('',(5.00596043934461E-16,1.,1.12027918221652E-15));
#38849=DIRECTION('center_axis',(5.57179392097266E-15,-1.12027918221652E-15,
1.));
#38850=DIRECTION('ref_axis',(-1.,5.00596043934455E-16,5.57179392097267E-15));
#38851=DIRECTION('',(5.00596043934461E-16,1.,1.12027918221652E-15));
#38852=DIRECTION('center_axis',(-5.00596043934461E-16,-1.,-1.12027918221652E-15));
#38853=DIRECTION('ref_axis',(-1.,5.00596043934455E-16,5.57179392097267E-15));
#38854=DIRECTION('',(5.00596043934461E-16,1.,1.12027918221652E-15));
#38855=DIRECTION('center_axis',(1.,-5.00596043934455E-16,-5.57179392097267E-15));
#38856=DIRECTION('ref_axis',(5.57179392097267E-15,-1.12027918221652E-15,
1.));
#48955=CARTESIAN_POINT('',(0.,0.,0.));
#48956=CARTESIAN_POINT('Origin',(263.115917770968,-85.47200726879,445.000000551893));
#48957=CARTESIAN_POINT('',(209.115917770968,-85.4720072687899,402.500000551893));
#48958=CARTESIAN_POINT('',(220.615917770968,-85.4720072687899,391.000000551893));
#48959=CARTESIAN_POINT('Origin',(220.615917770968,-85.4720072687899,402.500000551893));
#48960=CARTESIAN_POINT('',(305.615917770968,-85.47200726879,391.000000551893));
#48961=CARTESIAN_POINT('',(220.615917770968,-85.4720072687899,391.000000551893));
#48962=CARTESIAN_POINT('',(317.115917770968,-85.47200726879,402.500000551893));
#48963=CARTESIAN_POINT('Origin',(305.615917770968,-85.47200726879,402.500000551893));
#48964=CARTESIAN_POINT('',(317.115917770968,-85.4720072687901,487.500000551893));
#48965=CARTESIAN_POINT('',(317.115917770968,-85.47200726879,402.500000551893));
#48966=CARTESIAN_POINT('',(305.615917770968,-85.4720072687901,499.000000551893));
#48967=CARTESIAN_POINT('Origin',(305.615917770968,-85.4720072687901,487.500000551893));
#48968=CARTESIAN_POINT('',(220.615917770968,-85.47200726879,499.000000551893));
#48969=CARTESIAN_POINT('',(305.615917770968,-85.4720072687901,499.000000551893));
#48970=CARTESIAN_POINT('',(209.115917770968,-85.47200726879,487.500000551893));
#48971=CARTESIAN_POINT('Origin',(220.615917770968,-85.47200726879,487.500000551893));
#48972=CARTESIAN_POINT('',(209.115917770968,-85.47200726879,487.500000551893));
#48973=CARTESIAN_POINT('',(215.865917770968,-85.4720072687899,403.500000551893));
#48974=CARTESIAN_POINT('Origin',(221.615917770968,-85.4720072687899,403.500000551893));
#48975=CARTESIAN_POINT('',(298.865917770968,-85.47200726879,403.500000551893));
#48976=CARTESIAN_POINT('Origin',(304.615917770968,-85.47200726879,403.500000551893));
#48977=CARTESIAN_POINT('',(298.865917770968,-85.4720072687901,486.500000551893));
#48978=CARTESIAN_POINT('Origin',(304.615917770968,-85.4720072687901,486.500000551893));
#48979=CARTESIAN_POINT('',(215.865917770968,-85.47200726879,486.500000551893));
#48980=CARTESIAN_POINT('Origin',(221.615917770968,-85.47200726879,486.500000551893));
#48981=CARTESIAN_POINT('',(304.615917770968,-85.47200726879,415.000000551893));
#48982=CARTESIAN_POINT('',(293.115917770968,-85.47200726879,403.500000551893));
#48983=CARTESIAN_POINT('Origin',(304.615917770968,-85.47200726879,403.500000551893));
#48984=CARTESIAN_POINT('',(233.115917770968,-85.4720072687899,403.500000551893));
#48985=CARTESIAN_POINT('',(233.115917770968,-85.4720072687899,403.500000551893));
#48986=CARTESIAN_POINT('',(221.615917770968,-85.47200726879,415.000000551893));
#48987=CARTESIAN_POINT('Origin',(221.615917770968,-85.4720072687899,403.500000551893));
#48988=CARTESIAN_POINT('',(221.615917770968,-85.47200726879,475.000000551893));
#48989=CARTESIAN_POINT('',(221.615917770968,-85.47200726879,475.000000551893));
#48990=CARTESIAN_POINT('',(233.115917770968,-85.47200726879,486.500000551893));
#48991=CARTESIAN_POINT('Origin',(221.615917770968,-85.47200726879,486.500000551893));
#48992=CARTESIAN_POINT('',(293.115917770968,-85.4720072687901,486.500000551893));
#48993=CARTESIAN_POINT('',(293.115917770968,-85.4720072687901,486.500000551893));
#48994=CARTESIAN_POINT('',(304.615917770968,-85.4720072687901,475.000000551893));
#48995=CARTESIAN_POINT('Origin',(304.615917770968,-85.4720072687901,486.500000551893));
#48996=CARTESIAN_POINT('',(304.615917770968,-85.47200726879,415.000000551893));
#48997=CARTESIAN_POINT('Origin',(220.615917770968,-69.4720072687899,402.500000551893));
#48998=CARTESIAN_POINT('',(209.115917770967,-72.0120072687899,402.500000536626));
#48999=CARTESIAN_POINT('',(220.615917771658,-72.0120072687899,391.000000551893));
#49000=CARTESIAN_POINT('Origin',(220.615917770968,-72.0120072687899,402.500000551893));
#49001=CARTESIAN_POINT('',(220.615917770968,-85.4720072687899,391.000000551893));
#49002=CARTESIAN_POINT('',(209.115917770968,-85.4720072687899,402.500000551893));
#49003=CARTESIAN_POINT('Origin',(220.615917770968,-72.0120072687899,402.500000551893));
#49004=CARTESIAN_POINT('',(211.655917428536,-69.47200726879,402.500000528338));
#49005=CARTESIAN_POINT('Origin',(211.655917770968,-72.0120072687899,402.500000526873));
#49006=CARTESIAN_POINT('',(220.615917770968,-69.47200726879,393.540000209774));
#49007=CARTESIAN_POINT('Origin',(220.615917770968,-69.47200726879,402.500000551893));
#49008=CARTESIAN_POINT('Origin',(220.615917770968,-72.0120072687899,393.540000551893));
#49009=CARTESIAN_POINT('Origin',(220.367523674428,-72.0120072687899,393.540000551893));
#49010=CARTESIAN_POINT('',(227.022312716318,-69.4720072687899,393.540000551893));
#49011=CARTESIAN_POINT('',(220.615917770968,-69.4720072687899,393.540000551893));
#49012=CARTESIAN_POINT('',(227.022399311985,-72.0120048639452,391.000000934311));
#49013=CARTESIAN_POINT('Origin',(227.022312716318,-72.0120072687899,393.540000551893));
#49014=CARTESIAN_POINT('',(220.615917771658,-72.0120072687899,391.000000551893));
#49015=CARTESIAN_POINT('Origin',(263.115917770968,-69.47200726879,445.000000551893));
#49016=CARTESIAN_POINT('',(290.999730487759,-69.4720073199884,486.249685136186));
#49017=CARTESIAN_POINT('',(304.365591386209,-69.4720072899969,472.883807402065));
#49018=CARTESIAN_POINT('Origin',(263.115917770968,-69.4720072685233,445.000000551893));
#49019=CARTESIAN_POINT('',(299.209522825618,-69.4720072687901,496.460000551893));
#49020=CARTESIAN_POINT('',(290.999736208098,-69.4720072840695,486.249688664203));
#49021=CARTESIAN_POINT('',(305.615917770968,-69.4720072687901,496.460000894012));
#49022=CARTESIAN_POINT('',(305.615917770968,-69.4720072687901,496.460000551893));
#49023=CARTESIAN_POINT('',(314.5759181134,-69.4720072687901,487.500000575449));
#49024=CARTESIAN_POINT('Origin',(305.615917770968,-69.4720072687902,487.500000551893));
#49025=CARTESIAN_POINT('',(314.575917770968,-69.4720072687901,481.093605606543));
#49026=CARTESIAN_POINT('',(314.575917770968,-69.4720072687901,481.093605606543));
#49027=CARTESIAN_POINT('',(314.575917770968,-69.4720072687901,481.093605606543));
#49028=CARTESIAN_POINT('',(298.865917770968,-69.4720072687901,486.500000551893));
#49029=CARTESIAN_POINT('Origin',(304.615917770968,-69.4720072687901,486.500000551893));
#49030=CARTESIAN_POINT('Origin',(263.115917770968,-69.47200726879,445.000000551893));
#49031=CARTESIAN_POINT('',(304.365590681733,-69.4720072757894,417.116194305707));
#49032=CARTESIAN_POINT('',(290.999729934783,-69.4720072776403,403.750316697743));
#49033=CARTESIAN_POINT('Origin',(263.115917770968,-69.4720072684969,445.000000551893));
#49034=CARTESIAN_POINT('',(314.575917770968,-69.47200726879,408.906395497243));
#49035=CARTESIAN_POINT('',(304.365605883278,-69.4720072829853,417.116182114733));
#49036=CARTESIAN_POINT('',(314.575918113087,-69.47200726879,402.500000551893));
#49037=CARTESIAN_POINT('',(314.575917770968,-69.47200726879,402.500000551893));
#49038=CARTESIAN_POINT('',(305.615917794523,-69.47200726879,393.540000209461));
#49039=CARTESIAN_POINT('Origin',(305.615917770968,-69.4720072687901,402.500000551893));
#49040=CARTESIAN_POINT('',(299.209522825618,-69.47200726879,393.540000551893));
#49041=CARTESIAN_POINT('',(299.209522825618,-69.47200726879,393.540000551893));
#49042=CARTESIAN_POINT('',(299.209522825618,-69.47200726879,393.540000551893));
#49043=CARTESIAN_POINT('',(298.865917770968,-69.47200726879,403.500000551893));
#49044=CARTESIAN_POINT('Origin',(304.615917770968,-69.47200726879,403.500000551893));
#49045=CARTESIAN_POINT('Origin',(263.115917770968,-69.47200726879,445.000000551893));
#49046=CARTESIAN_POINT('',(235.232105054176,-69.4720073199883,403.750315967598));
#49047=CARTESIAN_POINT('',(221.866244155727,-69.4720072899968,417.116193701721));
#49048=CARTESIAN_POINT('Origin',(263.115917770968,-69.4720072685233,445.000000551893));
#49049=CARTESIAN_POINT('',(235.232099333838,-69.4720072840694,403.750312439583));
#49050=CARTESIAN_POINT('',(211.655917770968,-69.4720072687899,408.906395497243));
#49051=CARTESIAN_POINT('',(211.655917770968,-69.4720072687899,408.906395497243));
#49052=CARTESIAN_POINT('',(211.655917770968,-69.4720072687899,408.906395497243));
#49053=CARTESIAN_POINT('',(215.865917770968,-69.4720072687899,403.500000551893));
#49054=CARTESIAN_POINT('Origin',(221.615917770968,-69.4720072687899,403.500000551893));
#49055=CARTESIAN_POINT('Origin',(263.115917770968,-69.47200726879,445.000000551893));
#49056=CARTESIAN_POINT('',(221.866244860203,-69.4720072757895,472.883806798079));
#49057=CARTESIAN_POINT('',(235.232105607153,-69.4720072776404,486.249684406043));
#49058=CARTESIAN_POINT('Origin',(263.115917770968,-69.4720072684969,445.000000551893));
#49059=CARTESIAN_POINT('',(211.655917770968,-69.47200726879,481.093605606543));
#49060=CARTESIAN_POINT('',(221.866229658658,-69.4720072829853,472.883818989053));
#49061=CARTESIAN_POINT('',(211.655917428849,-69.4720072687901,487.500000551893));
#49062=CARTESIAN_POINT('',(211.655917770968,-69.47200726879,487.500000551893));
#49063=CARTESIAN_POINT('',(220.615917747413,-69.4720072687901,496.460000894325));
#49064=CARTESIAN_POINT('Origin',(220.615917770968,-69.4720072687901,487.500000551893));
#49065=CARTESIAN_POINT('',(227.022312716318,-69.47200726879,496.460000551893));
#49066=CARTESIAN_POINT('',(227.022312716318,-69.47200726879,496.460000551893));
#49067=CARTESIAN_POINT('',(227.022312716318,-69.47200726879,496.460000551893));
#49068=CARTESIAN_POINT('',(215.865917770968,-69.47200726879,486.500000551893));
#49069=CARTESIAN_POINT('Origin',(221.615917770968,-69.47200726879,486.500000551893));
#49070=CARTESIAN_POINT('Origin',(221.615917770968,-67.8720072687899,403.500000551893));
#49071=CARTESIAN_POINT('',(215.865917770968,-67.8720072687899,403.500000551893));
#49072=CARTESIAN_POINT('Origin',(304.615917770968,-67.87200726879,403.500000551893));
#49073=CARTESIAN_POINT('',(298.865917770968,-67.87200726879,403.500000551893));
#49074=CARTESIAN_POINT('Origin',(304.615917770968,-67.8720072687901,486.500000551893));
#49075=CARTESIAN_POINT('',(298.865917770968,-67.8720072687901,486.500000551893));
#49076=CARTESIAN_POINT('Origin',(221.615917770968,-67.87200726879,486.500000551893));
#49077=CARTESIAN_POINT('',(215.865917770968,-67.87200726879,486.500000551893));
#49078=CARTESIAN_POINT('Origin',(263.115917770968,-66.93200726879,445.000000551893));
#49079=CARTESIAN_POINT('',(302.261283577094,-66.93200726879,471.46134667694));
#49080=CARTESIAN_POINT('Origin',(304.365605883808,-66.9320073823691,472.883818948733));
#49081=CARTESIAN_POINT('',(289.577263857934,-66.932007268792,484.145366370259));
#49082=CARTESIAN_POINT('Origin',(263.115917770968,-66.93200726879,445.000000551893));
#49083=CARTESIAN_POINT('Origin',(290.999736208028,-66.93200726879,486.249688664283));
#49084=CARTESIAN_POINT('Ctrl Pts',(288.998285659208,-70.8410255423381,487.371976483543));
#49085=CARTESIAN_POINT('Ctrl Pts',(289.064861327528,-70.712722248464,487.348817061843));
#49086=CARTESIAN_POINT('Ctrl Pts',(289.246966153228,-70.4229586079247,487.284039301003));
#49087=CARTESIAN_POINT('Ctrl Pts',(289.613432565908,-70.0324228883725,487.143425190533));
#49088=CARTESIAN_POINT('Ctrl Pts',(290.085363845378,-69.7114497472353,486.941854741653));
#49089=CARTESIAN_POINT('Ctrl Pts',(290.593740217718,-69.5126381445131,486.698890965093));
#49090=CARTESIAN_POINT('Ctrl Pts',(290.971346420728,-69.4612407849915,486.497163873883));
#49091=CARTESIAN_POINT('Ctrl Pts',(291.171959587518,-69.464214633553,486.382871735513));
#49092=CARTESIAN_POINT('Ctrl Pts',(291.203406899448,-69.4654396674751,486.364779958613));
#49093=CARTESIAN_POINT('Ctrl Pts',(288.092412841418,-70.7821785594621,485.955461353113));
#49094=CARTESIAN_POINT('Ctrl Pts',(288.166834942358,-70.6531438863331,485.927338245653));
#49095=CARTESIAN_POINT('Ctrl Pts',(288.367773215418,-70.3684786785252,485.850444521383));
#49096=CARTESIAN_POINT('Ctrl Pts',(288.755212370428,-70.0112367740759,485.696202514793));
#49097=CARTESIAN_POINT('Ctrl Pts',(289.226188565798,-69.7468008290303,485.495309940943));
#49098=CARTESIAN_POINT('Ctrl Pts',(289.706503561258,-69.6062166524364,485.271875115773));
#49099=CARTESIAN_POINT('Ctrl Pts',(290.047780774728,-69.5867023581793,485.096173932863));
#49100=CARTESIAN_POINT('Ctrl Pts',(290.226195016768,-69.6011587121203,484.998161076463));
#49101=CARTESIAN_POINT('Ctrl Pts',(290.254102448988,-69.6040471487246,484.982674968233));
#49102=CARTESIAN_POINT('Ctrl Pts',(286.563889095188,-70.1428862842578,485.663027413833));
#49103=CARTESIAN_POINT('Ctrl Pts',(286.670561310298,-69.9482081499977,485.609927354613));
#49104=CARTESIAN_POINT('Ctrl Pts',(286.958062081058,-69.5204913988233,485.465578959453));
#49105=CARTESIAN_POINT('Ctrl Pts',(287.509285705738,-68.9908005466805,485.181938243533));
#49106=CARTESIAN_POINT('Ctrl Pts',(288.174844305588,-68.6071038509314,484.824524259113));
#49107=CARTESIAN_POINT('Ctrl Pts',(288.850431096308,-68.4105256300781,484.441925233693));
#49108=CARTESIAN_POINT('Ctrl Pts',(289.330116142288,-68.389499075236,484.152675406223));
#49109=CARTESIAN_POINT('Ctrl Pts',(289.581590656338,-68.4143084253991,483.994803323553));
#49110=CARTESIAN_POINT('Ctrl Pts',(289.620947839548,-68.4190995018021,483.969940141563));
#49111=CARTESIAN_POINT('Ctrl Pts',(285.486322930458,-69.372176498392,486.700075181433));
#49112=CARTESIAN_POINT('Ctrl Pts',(285.626997021668,-69.0930496471823,486.619528281213));
#49113=CARTESIAN_POINT('Ctrl Pts',(286.007989346758,-68.4746082940248,486.399765496033));
#49114=CARTESIAN_POINT('Ctrl Pts',(286.750769803908,-67.687850874675,485.961842661743));
#49115=CARTESIAN_POINT('Ctrl Pts',(287.669776998228,-67.092862159682,485.400645899203));
#49116=CARTESIAN_POINT('Ctrl Pts',(288.626813241638,-66.7653976675591,484.791983689493));
#49117=CARTESIAN_POINT('Ctrl Pts',(289.322427686498,-66.710525711832,484.329365258813));
#49118=CARTESIAN_POINT('Ctrl Pts',(289.690905404228,-66.7372867844731,484.077539521653));
#49119=CARTESIAN_POINT('Ctrl Pts',(289.748659863038,-66.742883356668,484.037902817103));
#49120=CARTESIAN_POINT('',(285.988731321319,-69.4720430411235,486.344876715169));
#49121=CARTESIAN_POINT('Ctrl Pts',(285.988756574376,-69.4718748783635,486.34485393706));
#49122=CARTESIAN_POINT('Ctrl Pts',(286.118744452923,-69.2047921984534,486.272949747314));
#49123=CARTESIAN_POINT('Ctrl Pts',(286.412224215766,-68.7100477492417,486.109000546669));
#49124=CARTESIAN_POINT('Ctrl Pts',(286.951205734338,-68.071986203272,485.799398096773));
#49125=CARTESIAN_POINT('Ctrl Pts',(287.559472514128,-67.566352173163,485.438326232773));
#49126=CARTESIAN_POINT('Ctrl Pts',(288.213563806918,-67.2011737721991,485.035967098023));
#49127=CARTESIAN_POINT('Ctrl Pts',(288.891014788688,-66.981639700943,484.603378736393));
#49128=CARTESIAN_POINT('Ctrl Pts',(289.347255309368,-66.932003603433,484.300842719953));
#49129=CARTESIAN_POINT('Ctrl Pts',(289.577263878948,-66.9320072687941,484.145366401723));
#49130=CARTESIAN_POINT('',(288.93249809502,-70.7420402776062,487.189112872311));
#49131=CARTESIAN_POINT('Origin',(287.218164767968,-69.4721762071729,488.567491527033));
#49132=CARTESIAN_POINT('Ctrl Pts',(288.93252952171,-70.7420200455039,487.189113576105));
#49133=CARTESIAN_POINT('Ctrl Pts',(288.988623498153,-70.6445951393942,487.169106682144));
#49134=CARTESIAN_POINT('Ctrl Pts',(289.050594887069,-70.5513567221658,487.146538078092));
#49135=CARTESIAN_POINT('Ctrl Pts',(289.141870461995,-70.4311536188864,487.112441714298));
#49136=CARTESIAN_POINT('Ctrl Pts',(289.166664996978,-70.4000028232925,487.103104730079));
#49137=CARTESIAN_POINT('Ctrl Pts',(289.288288528221,-70.2540727483778,487.056904492515));
#49138=CARTESIAN_POINT('Ctrl Pts',(289.393550533437,-70.1478860178951,487.015764059843));
#49139=CARTESIAN_POINT('Ctrl Pts',(289.510668415097,-70.0479200253442,486.968035327824));
#49140=CARTESIAN_POINT('Ctrl Pts',(289.516201545576,-70.0432370796359,486.96577616909));
#49141=CARTESIAN_POINT('Ctrl Pts',(289.628422450322,-69.9490612742506,486.919869119029));
#49142=CARTESIAN_POINT('Ctrl Pts',(289.740699614602,-69.8694544987993,486.872336831436));
#49143=CARTESIAN_POINT('Ctrl Pts',(289.900685400632,-69.7740400952016,486.801798814279));
#49144=CARTESIAN_POINT('Ctrl Pts',(289.945476928754,-69.7491804686929,486.781766067426));
#49145=CARTESIAN_POINT('Ctrl Pts',(290.069653334246,-69.6852131557637,486.725375784309));
#49146=CARTESIAN_POINT('Ctrl Pts',(290.14983936454,-69.6493657107357,486.688021219364));
#49147=CARTESIAN_POINT('Ctrl Pts',(290.316444820684,-69.5855318937613,486.608314250907));
#49148=CARTESIAN_POINT('Ctrl Pts',(290.402937085815,-69.5581670824828,486.565796223865));
#49149=CARTESIAN_POINT('Ctrl Pts',(290.531326493797,-69.525878339649,486.500878319984));
#49150=CARTESIAN_POINT('Ctrl Pts',(290.572982658775,-69.5166925224002,486.479536360681));
#49151=CARTESIAN_POINT('Ctrl Pts',(290.743416506245,-69.4843334129536,486.391078676298));
#49152=CARTESIAN_POINT('Ctrl Pts',(290.872510995065,-69.4720048208224,486.321377974098));
#49153=CARTESIAN_POINT('Ctrl Pts',(290.999733582907,-69.4720073298542,486.249690143456));
#49154=CARTESIAN_POINT('Origin',(263.115917770968,-85.47200726879,445.000000551893));
#49155=CARTESIAN_POINT('',(263.115917770968,-56.01200726879,492.250000551893));
#49156=CARTESIAN_POINT('',(262.857585971945,-56.01200726879,492.24929435277));
#49157=CARTESIAN_POINT('Origin',(263.115917770968,-56.01200726879,445.000000551893));
#49158=CARTESIAN_POINT('',(263.115917770968,-69.4720072687901,492.250000551893));
#49159=CARTESIAN_POINT('',(263.115917770968,-85.4720072687901,492.250000551893));
#49160=CARTESIAN_POINT('Origin',(263.115917770968,-69.47200726879,445.000000551893));
#49161=CARTESIAN_POINT('',(304.46086780848,-69.4721941921344,467.872700496303));
#49162=CARTESIAN_POINT('Ctrl Pts',(302.261283619528,-66.93200726879,471.461346659823));
#49163=CARTESIAN_POINT('Ctrl Pts',(302.418142881798,-66.932003845303,471.229292331673));
#49164=CARTESIAN_POINT('Ctrl Pts',(302.722783928448,-66.982389652618,470.769804097933));
#49165=CARTESIAN_POINT('Ctrl Pts',(303.158021100128,-67.205344908648,470.087868144283));
#49166=CARTESIAN_POINT('Ctrl Pts',(303.558526243438,-67.571638226744,469.436410965183));
#49167=CARTESIAN_POINT('Ctrl Pts',(303.916770751998,-68.074931862037,468.832754965133));
#49168=CARTESIAN_POINT('Ctrl Pts',(304.224868997438,-68.7101394690151,468.296382954193));
#49169=CARTESIAN_POINT('Ctrl Pts',(304.388818617838,-69.2046237434901,468.002914444963));
#49170=CARTESIAN_POINT('Ctrl Pts',(304.460794941428,-69.4719904999791,467.872796581653));
#49171=CARTESIAN_POINT('',(304.460780736566,-69.4720434315167,422.127162382352));
#49172=CARTESIAN_POINT('Origin',(263.115917770968,-69.47200726879,445.000000551893));
#49173=CARTESIAN_POINT('',(302.261283588757,-66.93200726879,418.53865446472));
#49174=CARTESIAN_POINT('Ctrl Pts',(304.460757971866,-69.4718531713743,422.127137633859));
#49175=CARTESIAN_POINT('Ctrl Pts',(304.388790543676,-69.2045390954083,421.997036357919));
#49176=CARTESIAN_POINT('Ctrl Pts',(304.224851420204,-68.7101031547398,421.703587571966));
#49177=CARTESIAN_POINT('Ctrl Pts',(303.916770755058,-68.074931865877,421.167246137583));
#49178=CARTESIAN_POINT('Ctrl Pts',(303.558526234868,-67.571638234798,420.563590126083));
#49179=CARTESIAN_POINT('Ctrl Pts',(303.158021102038,-67.20534489923,419.912132962153));
#49180=CARTESIAN_POINT('Ctrl Pts',(302.722783926568,-66.982389656305,419.230197003253));
#49181=CARTESIAN_POINT('Ctrl Pts',(302.418142881528,-66.932003845745,418.770708771203));
#49182=CARTESIAN_POINT('Ctrl Pts',(302.261283619518,-66.93200726879,418.538654443953));
#49183=CARTESIAN_POINT('',(289.577263929339,-66.9320072687885,405.854634796628));
#49184=CARTESIAN_POINT('Origin',(263.115917770968,-66.93200726879,445.000000551893));
#49185=CARTESIAN_POINT('',(285.988607027166,-69.4721792344465,403.655044784447));
#49186=CARTESIAN_POINT('Ctrl Pts',(289.577263854638,-66.932007268787,405.854634739443));
#49187=CARTESIAN_POINT('Ctrl Pts',(289.347343615378,-66.932005368643,405.699217182813));
#49188=CARTESIAN_POINT('Ctrl Pts',(288.891074071928,-66.981556806277,405.396653518833));
#49189=CARTESIAN_POINT('Ctrl Pts',(288.212152496378,-67.201691318908,404.963139413083));
#49190=CARTESIAN_POINT('Ctrl Pts',(287.557492638358,-67.567693344638,404.560478072123));
#49191=CARTESIAN_POINT('Ctrl Pts',(286.949480792468,-68.073737286196,404.199599095673));
#49192=CARTESIAN_POINT('Ctrl Pts',(286.411264535488,-68.7115153777147,403.890461337593));
#49193=CARTESIAN_POINT('Ctrl Pts',(286.118404220698,-69.2054638755325,403.726863292833));
#49194=CARTESIAN_POINT('Ctrl Pts',(285.988695062078,-69.47199135406,403.655113065203));
#49195=CARTESIAN_POINT('',(240.243104220617,-69.4720430411234,403.655124388617));
#49196=CARTESIAN_POINT('Origin',(263.115917770968,-69.47200726879,445.000000551893));
#49197=CARTESIAN_POINT('',(236.654571684002,-66.9320072687919,405.854634733527));
#49198=CARTESIAN_POINT('Ctrl Pts',(240.243078967561,-69.4718748783634,403.655147166726));
#49199=CARTESIAN_POINT('Ctrl Pts',(240.113091089014,-69.2047921984533,403.727051356473));
#49200=CARTESIAN_POINT('Ctrl Pts',(239.81961132617,-68.7100477492417,403.891000557117));
#49201=CARTESIAN_POINT('Ctrl Pts',(239.280629807598,-68.0719862032719,404.200603007013));
#49202=CARTESIAN_POINT('Ctrl Pts',(238.672363027808,-67.5663521731629,404.561674871013));
#49203=CARTESIAN_POINT('Ctrl Pts',(238.018271735018,-67.2011737721989,404.964034005763));
#49204=CARTESIAN_POINT('Ctrl Pts',(237.340820753248,-66.9816397009429,405.396622367393));
#49205=CARTESIAN_POINT('Ctrl Pts',(236.884580232568,-66.9320036034329,405.699158383833));
#49206=CARTESIAN_POINT('Ctrl Pts',(236.654571662988,-66.9320072687939,405.854634702063));
#49207=CARTESIAN_POINT('',(223.970551964843,-66.93200726879,418.538654426845));
#49208=CARTESIAN_POINT('Origin',(263.115917770968,-66.93200726879,445.000000551893));
#49209=CARTESIAN_POINT('',(221.770967733456,-69.4721941921343,422.127300607483));
#49210=CARTESIAN_POINT('Ctrl Pts',(223.970551922408,-66.9320072687899,418.538654443963));
#49211=CARTESIAN_POINT('Ctrl Pts',(223.813692660138,-66.9320038453029,418.770708772113));
#49212=CARTESIAN_POINT('Ctrl Pts',(223.509051613488,-66.9823896526179,419.230197005853));
#49213=CARTESIAN_POINT('Ctrl Pts',(223.073814441808,-67.2053449086479,419.912132959503));
#49214=CARTESIAN_POINT('Ctrl Pts',(222.673309298498,-67.5716382267429,420.563590138603));
#49215=CARTESIAN_POINT('Ctrl Pts',(222.315064789938,-68.0749318620369,421.167246138653));
#49216=CARTESIAN_POINT('Ctrl Pts',(222.006966544498,-68.7101394690148,421.703618149593));
#49217=CARTESIAN_POINT('Ctrl Pts',(221.843016924098,-69.20462374349,421.997086658823));
#49218=CARTESIAN_POINT('Ctrl Pts',(221.771040600508,-69.471990499979,422.127204522133));
#49219=CARTESIAN_POINT('',(221.771098592854,-69.4723526686334,467.87293717337));
#49220=CARTESIAN_POINT('Origin',(263.115917770968,-69.47200726879,445.000000551893));
#49221=CARTESIAN_POINT('',(223.970551953179,-66.93200726879,471.461346639066));
#49222=CARTESIAN_POINT('Ctrl Pts',(221.771077570127,-69.4718531714348,467.872863470021));
#49223=CARTESIAN_POINT('Ctrl Pts',(221.84304499834,-69.2045390954037,468.002964746004));
#49224=CARTESIAN_POINT('Ctrl Pts',(222.006984121657,-68.7101031548514,468.296413531676));
#49225=CARTESIAN_POINT('Ctrl Pts',(222.315064786898,-68.074931865861,468.832754966233));
#49226=CARTESIAN_POINT('Ctrl Pts',(222.673309307068,-67.571638234802,469.436410977693));
#49227=CARTESIAN_POINT('Ctrl Pts',(223.073814439898,-67.205344899229,470.087868141633));
#49228=CARTESIAN_POINT('Ctrl Pts',(223.509051615368,-66.982389656305,470.769804100533));
#49229=CARTESIAN_POINT('Ctrl Pts',(223.813692660408,-66.932003845745,471.229292332583));
#49230=CARTESIAN_POINT('Ctrl Pts',(223.970551922418,-66.93200726879,471.461346659833));
#49231=CARTESIAN_POINT('',(236.654571612597,-66.9320072687885,484.145366307158));
#49232=CARTESIAN_POINT('Origin',(263.115917770968,-66.93200726879,445.000000551893));
#49233=CARTESIAN_POINT('',(240.24303782791,-69.4723069190014,486.344850841488));
#49234=CARTESIAN_POINT('Ctrl Pts',(236.654571687298,-66.932007268787,484.145366364343));
#49235=CARTESIAN_POINT('Ctrl Pts',(236.884491926558,-66.932005368643,484.300783920973));
#49236=CARTESIAN_POINT('Ctrl Pts',(237.340761470018,-66.981556806277,484.603347584953));
#49237=CARTESIAN_POINT('Ctrl Pts',(238.019683045558,-67.201691318908,485.036861690703));
#49238=CARTESIAN_POINT('Ctrl Pts',(238.674342903578,-67.567693344638,485.439523031663));
#49239=CARTESIAN_POINT('Ctrl Pts',(239.282354749468,-68.073737286197,485.800402008113));
#49240=CARTESIAN_POINT('Ctrl Pts',(239.820546721509,-68.7114866004303,486.10952581754));
#49241=CARTESIAN_POINT('Ctrl Pts',(240.113391678348,-69.2053970132659,486.27311566556));
#49242=CARTESIAN_POINT('Ctrl Pts',(240.243087805294,-69.4718831208831,486.344858900952));
#49243=CARTESIAN_POINT('Origin',(263.115917770968,-69.47200726879,445.000000551893));
#49244=CARTESIAN_POINT('Origin',(263.115917770968,-56.01200726879,445.000000551893));
#49245=CARTESIAN_POINT('Origin',(263.115917770968,-69.47200726879,445.000000551893));
#49246=CARTESIAN_POINT('',(287.218198108558,-72.0120072687901,488.567467571773));
#49247=CARTESIAN_POINT('',(239.013637433378,-72.01200726879,488.567467571773));
#49248=CARTESIAN_POINT('Origin',(263.115917770968,-72.01200726879,445.000000551893));
#49249=CARTESIAN_POINT('Origin',(287.218198108558,-69.4720072687901,488.567467571773));
#49250=CARTESIAN_POINT('Origin',(239.013637433378,-69.47200726879,488.567467571773));
#49251=CARTESIAN_POINT('Origin',(263.115917770968,-72.01200726879,445.000000551893));
#49252=CARTESIAN_POINT('',(232.66750323717,-72.0120085167185,496.460000513384));
#49253=CARTESIAN_POINT('',(232.667503020318,-72.012008100742,496.460000551893));
#49254=CARTESIAN_POINT('',(293.564332521699,-72.0120076847427,496.460000551919));
#49255=CARTESIAN_POINT('',(293.564332521618,-72.0120081006951,496.460000551893));
#49256=CARTESIAN_POINT('',(287.218030147038,-72.0120072687901,488.567258682123));
#49257=CARTESIAN_POINT('Origin',(263.115917770968,-72.01200726879,445.000000551893));
#49258=CARTESIAN_POINT('',(306.683384791277,-72.0120072687908,469.102280888707));
#49259=CARTESIAN_POINT('',(306.683384791312,-72.0120072687919,420.897720215143));
#49260=CARTESIAN_POINT('Origin',(263.115917770968,-72.01200726879,445.000000551893));
#49261=CARTESIAN_POINT('',(314.575917732466,-72.0120093486708,475.448415085728));
#49262=CARTESIAN_POINT('',(314.575917770968,-72.0120081007421,475.448415302543));
#49263=CARTESIAN_POINT('',(314.575917770971,-72.012008516648,414.551585801181));
#49264=CARTESIAN_POINT('',(314.575917770968,-72.012008100695,414.551585801243));
#49265=CARTESIAN_POINT('',(306.683313170078,-72.01200726879,420.897777802283));
#49266=CARTESIAN_POINT('Origin',(263.115917770968,-72.01200726879,445.000000551893));
#49267=CARTESIAN_POINT('',(239.013637433378,-72.0120072687899,401.432533532013));
#49268=CARTESIAN_POINT('',(287.218198108558,-72.01200726879,401.432533532013));
#49269=CARTESIAN_POINT('Origin',(263.115917770968,-72.01200726879,445.000000551893));
#49270=CARTESIAN_POINT('',(293.564332304803,-72.0120093486707,393.540000590395));
#49271=CARTESIAN_POINT('',(293.564332521618,-72.012008100742,393.540000551893));
#49272=CARTESIAN_POINT('',(232.667503020229,-72.0120085166479,393.540000551878));
#49273=CARTESIAN_POINT('',(232.667503020318,-72.0120081006949,393.540000551893));
#49274=CARTESIAN_POINT('',(239.013805394898,-72.0120072687899,401.432742421663));
#49275=CARTESIAN_POINT('Origin',(263.115917770968,-72.01200726879,445.000000551893));
#49276=CARTESIAN_POINT('',(219.548450750635,-72.0120072687917,420.897720215124));
#49277=CARTESIAN_POINT('',(219.548450750735,-72.0120072687907,469.102280888843));
#49278=CARTESIAN_POINT('Origin',(263.115917770968,-72.01200726879,445.000000551893));
#49279=CARTESIAN_POINT('',(211.655917809477,-72.0120085167184,414.551586018095));
#49280=CARTESIAN_POINT('',(211.655917770968,-72.0120081007419,414.551585801243));
#49281=CARTESIAN_POINT('',(211.655917770966,-72.012008516648,475.448415302606));
#49282=CARTESIAN_POINT('',(211.655917770968,-72.012008100695,475.448415302543));
#49283=CARTESIAN_POINT('',(219.548478072158,-72.01200726879,469.102258921483));
#49284=CARTESIAN_POINT('Origin',(208.622849682388,-69.4720072687899,390.820344809323));
#49285=CARTESIAN_POINT('Origin',(287.218198108558,-69.4720072687901,488.567467571773));
#49286=CARTESIAN_POINT('',(297.495237745731,-70.7420027751341,497.838375097668));
#49287=CARTESIAN_POINT('Ctrl Pts',(297.495223246486,-70.7420072386772,497.838360765429));
#49288=CARTESIAN_POINT('Ctrl Pts',(297.430584327513,-70.8046621666009,497.815698843203));
#49289=CARTESIAN_POINT('Ctrl Pts',(297.360281447534,-70.8666202157765,497.791051170732));
#49290=CARTESIAN_POINT('Ctrl Pts',(297.28423434323,-70.927488967184,497.764391959688));
#49291=CARTESIAN_POINT('Ctrl Pts',(297.249478309544,-70.955307993216,497.752207821376));
#49292=CARTESIAN_POINT('Ctrl Pts',(297.213522928337,-70.9828991882139,497.739603111736));
#49293=CARTESIAN_POINT('Ctrl Pts',(297.176363170917,-71.0102237238982,497.726573251284));
#49294=CARTESIAN_POINT('Ctrl Pts',(297.099408625323,-71.0668104018838,497.699589571629));
#49295=CARTESIAN_POINT('Ctrl Pts',(297.017285377873,-71.1222548073893,497.670785396027));
#49296=CARTESIAN_POINT('Ctrl Pts',(296.930099031586,-71.17617908362,497.640217390304));
#49297=CARTESIAN_POINT('Ctrl Pts',(296.883067947229,-71.2052675509352,497.623728037131));
#49298=CARTESIAN_POINT('Ctrl Pts',(296.834564258945,-71.233913619238,497.606724878083));
#49299=CARTESIAN_POINT('Ctrl Pts',(296.784609466707,-71.2620580049096,497.589212848827));
#49300=CARTESIAN_POINT('Ctrl Pts',(296.710034719059,-71.304073202354,497.56307010848));
#49301=CARTESIAN_POINT('Ctrl Pts',(296.632228985522,-71.3449729686995,497.535790957057));
#49302=CARTESIAN_POINT('Ctrl Pts',(296.550979327238,-71.3847000761761,497.507298519727));
#49303=CARTESIAN_POINT('Ctrl Pts',(296.476907750018,-71.4209174532253,497.481323274828));
#49304=CARTESIAN_POINT('Ctrl Pts',(296.399973458015,-71.4561599907446,497.454339993113));
#49305=CARTESIAN_POINT('Ctrl Pts',(296.320005933237,-71.4903483914338,497.426297806313));
#49306=CARTESIAN_POINT('Ctrl Pts',(296.236163687569,-71.5261933459647,497.396896872354));
#49307=CARTESIAN_POINT('Ctrl Pts',(296.148991000274,-71.5608777497719,497.366328831849));
#49308=CARTESIAN_POINT('Ctrl Pts',(296.058184783034,-71.5942905948271,497.334485472522));
#49309=CARTESIAN_POINT('Ctrl Pts',(295.974225761459,-71.6251839616489,497.305043245171));
#49310=CARTESIAN_POINT('Ctrl Pts',(295.887160058519,-71.6549900460394,497.274511147639));
#49311=CARTESIAN_POINT('Ctrl Pts',(295.796743844254,-71.6835702845246,497.24280707608));
#49312=CARTESIAN_POINT('Ctrl Pts',(295.789370038573,-71.685901117845,497.240221481617));
#49313=CARTESIAN_POINT('Ctrl Pts',(295.781973948109,-71.6882237691193,497.237628092557));
#49314=CARTESIAN_POINT('Ctrl Pts',(295.774555440656,-71.6905381475854,497.235026864326));
#49315=CARTESIAN_POINT('Ctrl Pts',(295.684394659189,-71.7186659310274,497.203412854148));
#49316=CARTESIAN_POINT('Ctrl Pts',(295.590927640836,-71.7455720207983,497.170636985462));
#49317=CARTESIAN_POINT('Ctrl Pts',(295.493955551593,-71.7710584862261,497.136633017367));
#49318=CARTESIAN_POINT('Ctrl Pts',(295.400012919925,-71.7957487414619,497.103691350595));
#49319=CARTESIAN_POINT('Ctrl Pts',(295.302780415339,-71.8191066957974,497.069597425559));
#49320=CARTESIAN_POINT('Ctrl Pts',(295.20208695446,-71.8409047899498,497.034283224832));
#49321=CARTESIAN_POINT('Ctrl Pts',(295.179882407108,-71.8457116245701,497.026495868678));
#49322=CARTESIAN_POINT('Ctrl Pts',(295.157509613646,-71.8504424182202,497.018649132406));
#49323=CARTESIAN_POINT('Ctrl Pts',(295.13496683554,-71.8550944056927,497.010742209453));
#49324=CARTESIAN_POINT('Ctrl Pts',(295.029517193622,-71.876855273447,496.973755543918));
#49325=CARTESIAN_POINT('Ctrl Pts',(294.920346256765,-71.8968900354862,496.935453348788));
#49326=CARTESIAN_POINT('Ctrl Pts',(294.807768064222,-71.9148342843373,496.895973288881));
#49327=CARTESIAN_POINT('Ctrl Pts',(294.69684542964,-71.9325146477646,496.857073816796));
#49328=CARTESIAN_POINT('Ctrl Pts',(294.582615070484,-71.9481650394229,496.817030824154));
#49329=CARTESIAN_POINT('Ctrl Pts',(294.465415417878,-71.9614508713659,496.775945401434));
#49330=CARTESIAN_POINT('Ctrl Pts',(294.44178868109,-71.9641292142394,496.767662830225));
#49331=CARTESIAN_POINT('Ctrl Pts',(294.418041395273,-71.9667115210617,496.759337795346));
#49332=CARTESIAN_POINT('Ctrl Pts',(294.394176519811,-71.9691951485018,496.750970974903));
#49333=CARTESIAN_POINT('Ctrl Pts',(294.286409353994,-71.9804105219317,496.713188731813));
#49334=CARTESIAN_POINT('Ctrl Pts',(294.176244821695,-71.9896168634752,496.674554011708));
#49335=CARTESIAN_POINT('Ctrl Pts',(294.063676027197,-71.9965893765212,496.635082677501));
#49336=CARTESIAN_POINT('Ctrl Pts',(293.954872495805,-72.0033286691063,496.596931602244));
#49337=CARTESIAN_POINT('Ctrl Pts',(293.843822487108,-72.0079808733766,496.557999236117));
#49338=CARTESIAN_POINT('Ctrl Pts',(293.730541954548,-72.0103037875458,496.518282068601));
#49339=CARTESIAN_POINT('Ctrl Pts',(293.675660579299,-72.0114291770661,496.499040167764));
#49340=CARTESIAN_POINT('Ctrl Pts',(293.620256039227,-72.0120072687892,496.479613764687));
#49341=CARTESIAN_POINT('Ctrl Pts',(293.564332521698,-72.0120072687901,496.460000551921));
#49342=CARTESIAN_POINT('',(288.932517128318,-70.742010863496,487.189123540753));
#49343=CARTESIAN_POINT('Origin',(287.218198108558,-69.4720072687901,488.567467571773));
#49344=CARTESIAN_POINT('Origin',(214.070843635538,-72.0120072687899,390.575096505143));
#49345=CARTESIAN_POINT('Origin',(299.209522825618,-72.0120072687901,496.460000551893));
#49346=CARTESIAN_POINT('Origin',(299.209522825618,-72.0120072687901,496.460000551893));
#49347=CARTESIAN_POINT('',(299.209436229951,-72.0120048639454,499.000000169476));
#49348=CARTESIAN_POINT('Origin',(299.209530492038,-72.0119940551321,496.460000551893));
#49349=CARTESIAN_POINT('Origin',(299.209522825618,-72.0120072687901,496.460000551893));
#49350=CARTESIAN_POINT('Origin',(305.864311867508,-72.0120072687901,496.460000551893));
#49351=CARTESIAN_POINT('',(305.615917770278,-72.0120072687901,499.000000551893));
#49352=CARTESIAN_POINT('',(305.615917770278,-72.0120072687901,499.000000551893));
#49353=CARTESIAN_POINT('Origin',(305.615917770968,-72.0120072687901,496.460000551893));
#49354=CARTESIAN_POINT('Origin',(305.615917770968,-72.0120072687901,487.500000551893));
#49355=CARTESIAN_POINT('',(317.115917770969,-72.0120072687902,487.50000056716));
#49356=CARTESIAN_POINT('Origin',(305.615917770968,-72.0120072687901,487.500000551893));
#49357=CARTESIAN_POINT('Origin',(314.575917770968,-72.0120072687901,487.500000576913));
#49358=CARTESIAN_POINT('Origin',(305.615917770968,-69.4720072687901,487.500000551893));
#49359=CARTESIAN_POINT('',(305.615917770968,-85.4720072687901,499.000000551893));
#49360=CARTESIAN_POINT('',(317.115917770968,-85.4720072687901,487.500000551893));
#49361=CARTESIAN_POINT('Origin',(317.115917770968,-69.4720072687901,487.500000551893));
#49362=CARTESIAN_POINT('',(317.115917770968,-72.01200726879,402.500000552583));
#49363=CARTESIAN_POINT('',(317.115917388551,-72.0120048639453,408.90648209291));
#49364=CARTESIAN_POINT('',(317.115917770968,-72.01200726879,402.500000552583));
#49365=CARTESIAN_POINT('',(317.115921985178,-74.552007268779,414.551585800843));
#49366=CARTESIAN_POINT('Ctrl Pts',(317.115917292418,-72.012007955791,408.906503863893));
#49367=CARTESIAN_POINT('Ctrl Pts',(317.115920597578,-72.19552121824,409.042444578523));
#49368=CARTESIAN_POINT('Ctrl Pts',(317.115916447358,-72.553339671846,409.346292243203));
#49369=CARTESIAN_POINT('Ctrl Pts',(317.115918163698,-73.060368305257,409.910077792133));
#49370=CARTESIAN_POINT('Ctrl Pts',(317.115917523658,-73.517848719505,410.575025306713));
#49371=CARTESIAN_POINT('Ctrl Pts',(317.115918367468,-73.920471429642,411.354781495243));
#49372=CARTESIAN_POINT('Ctrl Pts',(317.115915632288,-74.254566710336,412.270129474193));
#49373=CARTESIAN_POINT('Ctrl Pts',(317.115925729188,-74.490207324085,413.339593273333));
#49374=CARTESIAN_POINT('Ctrl Pts',(317.115900627578,-74.551992485447,414.132916486413));
#49375=CARTESIAN_POINT('Ctrl Pts',(317.115921985178,-74.552007268779,414.551585800843));
#49376=CARTESIAN_POINT('',(317.115921689795,-74.5520072687783,475.448415303017));
#49377=CARTESIAN_POINT('',(317.115921985178,-74.552007268779,414.551585800843));
#49378=CARTESIAN_POINT('',(317.115917387258,-72.0120079573944,481.093518686536));
#49379=CARTESIAN_POINT('Ctrl Pts',(317.115921985308,-74.5520072687791,475.448415303033));
#49380=CARTESIAN_POINT('Ctrl Pts',(317.115900627238,-74.5519924846921,475.867084617403));
#49381=CARTESIAN_POINT('Ctrl Pts',(317.115925729348,-74.4902073241181,476.660407830253));
#49382=CARTESIAN_POINT('Ctrl Pts',(317.115915632248,-74.254566710358,477.729871629363));
#49383=CARTESIAN_POINT('Ctrl Pts',(317.115918367468,-73.9204714300721,478.645219608463));
#49384=CARTESIAN_POINT('Ctrl Pts',(317.115917523708,-73.5178487189331,479.424975796243));
#49385=CARTESIAN_POINT('Ctrl Pts',(317.115918163528,-73.0603683068281,480.089923312253));
#49386=CARTESIAN_POINT('Ctrl Pts',(317.115916447978,-72.5533396705431,480.653708859803));
#49387=CARTESIAN_POINT('Ctrl Pts',(317.115920596228,-72.1955212187221,480.957556521343));
#49388=CARTESIAN_POINT('Ctrl Pts',(317.115917292588,-72.0120079573931,481.093497241393));
#49389=CARTESIAN_POINT('',(317.115917292588,-72.0120079573931,481.093497241393));
#49390=CARTESIAN_POINT('',(317.115917770968,-85.47200726879,402.500000551893));
#49391=CARTESIAN_POINT('Origin',(314.575917770968,-72.01200726879,402.251606455353));
#49392=CARTESIAN_POINT('Origin',(314.575917770968,-72.01200726879,408.906395497243));
#49393=CARTESIAN_POINT('Origin',(314.575917770968,-72.01200726879,402.500000551893));
#49394=CARTESIAN_POINT('Origin',(305.615917770968,-72.01200726879,402.500000551893));
#49395=CARTESIAN_POINT('',(305.615917786235,-72.0120072687901,391.000000551892));
#49396=CARTESIAN_POINT('Origin',(305.615917770968,-72.01200726879,402.500000551893));
#49397=CARTESIAN_POINT('Origin',(305.615917795988,-72.01200726879,393.540000551893));
#49398=CARTESIAN_POINT('Origin',(305.615917770968,-69.47200726879,402.500000551893));
#49399=CARTESIAN_POINT('',(305.615917770968,-85.47200726879,391.000000551893));
#49400=CARTESIAN_POINT('Origin',(305.615917770968,-69.47200726879,391.000000551893));
#49401=CARTESIAN_POINT('',(293.564332522092,-74.5520072687782,390.999996633066));
#49402=CARTESIAN_POINT('',(299.209435905611,-72.0120079573942,391.000000935603));
#49403=CARTESIAN_POINT('Ctrl Pts',(293.564332522108,-74.5520072687789,390.999996337553));
#49404=CARTESIAN_POINT('Ctrl Pts',(293.983001836478,-74.551992484692,391.000017695623));
#49405=CARTESIAN_POINT('Ctrl Pts',(294.776325049328,-74.4902073241179,390.999992593513));
#49406=CARTESIAN_POINT('Ctrl Pts',(295.845788848438,-74.2545667103579,391.000002690613));
#49407=CARTESIAN_POINT('Ctrl Pts',(296.761136827538,-73.920471430072,390.999999955393));
#49408=CARTESIAN_POINT('Ctrl Pts',(297.540893015318,-73.517848718933,391.000000799153));
#49409=CARTESIAN_POINT('Ctrl Pts',(298.205840531328,-73.060368306828,391.000000159333));
#49410=CARTESIAN_POINT('Ctrl Pts',(298.769626078878,-72.553339670543,391.000001874883));
#49411=CARTESIAN_POINT('Ctrl Pts',(299.073473740418,-72.195521218722,390.999997726633));
#49412=CARTESIAN_POINT('Ctrl Pts',(299.209414460468,-72.012007957393,391.000001030273));
#49413=CARTESIAN_POINT('',(299.209414460468,-72.012007957393,391.000001030273));
#49414=CARTESIAN_POINT('',(232.667503019918,-74.5520072687789,390.999996337683));
#49415=CARTESIAN_POINT('Ctrl Pts',(227.022421082968,-72.0120079557909,391.000001030443));
#49416=CARTESIAN_POINT('Ctrl Pts',(227.158361797598,-72.1955212182399,390.999997725283));
#49417=CARTESIAN_POINT('Ctrl Pts',(227.462209462278,-72.5533396718459,391.000001875503));
#49418=CARTESIAN_POINT('Ctrl Pts',(228.025995011208,-73.0603683052569,391.000000159163));
#49419=CARTESIAN_POINT('Ctrl Pts',(228.690942525788,-73.5178487195049,391.000000799203));
#49420=CARTESIAN_POINT('Ctrl Pts',(229.470698714318,-73.9204714296419,390.999999955393));
#49421=CARTESIAN_POINT('Ctrl Pts',(230.386046693268,-74.2545667103359,391.000002690573));
#49422=CARTESIAN_POINT('Ctrl Pts',(231.455510492408,-74.4902073240849,390.999992593673));
#49423=CARTESIAN_POINT('Ctrl Pts',(232.248833705488,-74.5519924854469,391.000017695283));
#49424=CARTESIAN_POINT('Ctrl Pts',(232.667503019918,-74.5520072687789,390.999996337683));
#49425=CARTESIAN_POINT('',(232.667503019918,-74.5520072687789,390.999996337683));
#49426=CARTESIAN_POINT('Ctrl Pts',(293.403620000158,-74.713507444107,391.005206331223));
#49427=CARTESIAN_POINT('Ctrl Pts',(293.523253662578,-74.7444877320719,391.007066101423));
#49428=CARTESIAN_POINT('Ctrl Pts',(294.096491996468,-74.8792972330759,391.018187674123));
#49429=CARTESIAN_POINT('Ctrl Pts',(295.116742986068,-75.0078404229239,391.055676766553));
#49430=CARTESIAN_POINT('Ctrl Pts',(296.436962017788,-74.9488215722139,391.135288071793));
#49431=CARTESIAN_POINT('Ctrl Pts',(297.629286318478,-74.6941844595169,391.229364066743));
#49432=CARTESIAN_POINT('Ctrl Pts',(298.687681546088,-74.2773859025649,391.328484148293));
#49433=CARTESIAN_POINT('Ctrl Pts',(299.613647008578,-73.717781829922,391.426026814723));
#49434=CARTESIAN_POINT('Ctrl Pts',(300.228909735688,-73.1791351904629,391.496377994003));
#49435=CARTESIAN_POINT('Ctrl Pts',(300.530920362218,-72.841170440473,391.532173125083));
#49436=CARTESIAN_POINT('Ctrl Pts',(300.593570177078,-72.767200936835,391.539646373643));
#49437=CARTESIAN_POINT('Ctrl Pts',(293.435266749438,-73.0348243119389,390.897237502753));
#49438=CARTESIAN_POINT('Ctrl Pts',(293.531207702328,-73.0665839015929,390.880070293753));
#49439=CARTESIAN_POINT('Ctrl Pts',(293.992363219048,-73.2090046443279,390.801058739933));
#49440=CARTESIAN_POINT('Ctrl Pts',(294.824652130898,-73.3818065881169,390.686408027683));
#49441=CARTESIAN_POINT('Ctrl Pts',(295.922404003618,-73.4353515830609,390.584022189883));
#49442=CARTESIAN_POINT('Ctrl Pts',(296.929923102608,-73.326904152345,390.525172261023));
#49443=CARTESIAN_POINT('Ctrl Pts',(297.836986340198,-73.078553798327,390.497473304713));
#49444=CARTESIAN_POINT('Ctrl Pts',(298.640699611108,-72.7034694849989,390.491103395363));
#49445=CARTESIAN_POINT('Ctrl Pts',(299.180855751788,-72.31828963445,390.496606056823));
#49446=CARTESIAN_POINT('Ctrl Pts',(299.447631606278,-72.069395060257,390.501676649803));
#49447=CARTESIAN_POINT('Ctrl Pts',(299.503042114118,-72.014632724146,390.502823399773));
#49448=CARTESIAN_POINT('Ctrl Pts',(293.457348103978,-71.8635323633289,392.104816764133));
#49449=CARTESIAN_POINT('Ctrl Pts',(293.537031632768,-71.8812991757079,392.074367240203));
#49450=CARTESIAN_POINT('Ctrl Pts',(293.918365156668,-71.960042879052,391.931270597373));
#49451=CARTESIAN_POINT('Ctrl Pts',(294.593238217918,-72.047682887232,391.699013943113));
#49452=CARTESIAN_POINT('Ctrl Pts',(295.459642360368,-72.0525390584189,391.438419217373));
#49453=CARTESIAN_POINT('Ctrl Pts',(296.236766415788,-71.958291489615,391.232931397543));
#49454=CARTESIAN_POINT('Ctrl Pts',(296.922378360948,-71.779984113589,391.072990588673));
#49455=CARTESIAN_POINT('Ctrl Pts',(297.518836711668,-71.526452518351,390.950035877043));
#49456=CARTESIAN_POINT('Ctrl Pts',(297.913123545478,-71.274222914498,390.878004465333));
#49457=CARTESIAN_POINT('Ctrl Pts',(298.106123060458,-71.1135155794619,390.845098548043));
#49458=CARTESIAN_POINT('Ctrl Pts',(298.146136149308,-71.0782444347639,390.838373797913));
#49459=CARTESIAN_POINT('Ctrl Pts',(293.454354624918,-72.0223202985269,393.779768035813));
#49460=CARTESIAN_POINT('Ctrl Pts',(293.536634858248,-72.021150461685,393.751110055733));
#49461=CARTESIAN_POINT('Ctrl Pts',(293.926472357468,-72.009654141941,393.614988263533));
#49462=CARTESIAN_POINT('Ctrl Pts',(294.585041091708,-71.942527322552,393.382263256273));
#49463=CARTESIAN_POINT('Ctrl Pts',(295.373710291988,-71.7716399178189,393.098370205453));
#49464=CARTESIAN_POINT('Ctrl Pts',(296.036673675948,-71.5496287323249,392.855527631373));
#49465=CARTESIAN_POINT('Ctrl Pts',(296.586257353848,-71.293762522114,392.650805810713));
#49466=CARTESIAN_POINT('Ctrl Pts',(297.036029175858,-71.0134407520789,392.480480571413));
#49467=CARTESIAN_POINT('Ctrl Pts',(297.316139250318,-70.780263637391,392.372687692493));
#49468=CARTESIAN_POINT('Ctrl Pts',(297.448639673388,-70.644919903199,392.321227125813));
#49469=CARTESIAN_POINT('Ctrl Pts',(297.475912026518,-70.6157338063319,392.310614635863));
#49470=CARTESIAN_POINT('',(297.495234411945,-70.7420091884828,392.161623914219));
#49471=CARTESIAN_POINT('Ctrl Pts',(293.564332521712,-72.0120105965991,393.540000551893));
#49472=CARTESIAN_POINT('Ctrl Pts',(293.610180177156,-72.0120088645519,393.523921124626));
#49473=CARTESIAN_POINT('Ctrl Pts',(293.655679608989,-72.0116188869948,393.507964757136));
#49474=CARTESIAN_POINT('Ctrl Pts',(293.700828127475,-72.0108586572667,393.492132222862));
#49475=CARTESIAN_POINT('Ctrl Pts',(293.821427560535,-72.0088279533303,393.449840809511));
#49476=CARTESIAN_POINT('Ctrl Pts',(293.939519908192,-72.0041577141726,393.408434113532));
#49477=CARTESIAN_POINT('Ctrl Pts',(294.05507958132,-71.9971271823479,393.367917803027));
#49478=CARTESIAN_POINT('Ctrl Pts',(294.170639254449,-71.9900966505231,393.327401492523));
#49479=CARTESIAN_POINT('Ctrl Pts',(294.283666851026,-71.9807057284239,393.28777534827));
#49480=CARTESIAN_POINT('Ctrl Pts',(294.394177386595,-71.9692011295368,393.24903082564));
#49481=CARTESIAN_POINT('Ctrl Pts',(294.469689910043,-71.9613399668995,393.222556456852));
#49482=CARTESIAN_POINT('Ctrl Pts',(294.544023221346,-71.9524908559285,393.196494275085));
#49483=CARTESIAN_POINT('Ctrl Pts',(294.61708943307,-71.9427410029954,393.170874910482));
#49484=CARTESIAN_POINT('Ctrl Pts',(294.720519831422,-71.9289393955364,393.134608885136));
#49485=CARTESIAN_POINT('Ctrl Pts',(294.821408954925,-71.9133317336542,393.099230965762));
#49486=CARTESIAN_POINT('Ctrl Pts',(294.919510626567,-71.8961610227596,393.06482701592));
#49487=CARTESIAN_POINT('Ctrl Pts',(294.992918738488,-71.8833124194074,393.039083020347));
#49488=CARTESIAN_POINT('Ctrl Pts',(295.064767002146,-71.8695891220288,393.013884055383));
#49489=CARTESIAN_POINT('Ctrl Pts',(295.13496867765,-71.8551008150858,392.989260375731));
#49490=CARTESIAN_POINT('Ctrl Pts',(295.23044268125,-71.8353967744157,392.955772267892));
#49491=CARTESIAN_POINT('Ctrl Pts',(295.322858820816,-71.8142817745928,392.923362377343));
#49492=CARTESIAN_POINT('Ctrl Pts',(295.412369258352,-71.7919537135011,392.891974213068));
#49493=CARTESIAN_POINT('Ctrl Pts',(295.508894470344,-71.767875841807,392.858126213951));
#49494=CARTESIAN_POINT('Ctrl Pts',(295.602039818024,-71.7423873942477,392.825466660148));
#49495=CARTESIAN_POINT('Ctrl Pts',(295.691974537143,-71.7156824432709,392.793932532312));
#49496=CARTESIAN_POINT('Ctrl Pts',(295.719807600318,-71.707417775355,392.784173327181));
#49497=CARTESIAN_POINT('Ctrl Pts',(295.747333405952,-71.6990363146507,392.774521827672));
#49498=CARTESIAN_POINT('Ctrl Pts',(295.774557578644,-71.6905430693269,392.764975958906));
#49499=CARTESIAN_POINT('Ctrl Pts',(295.865554257107,-71.6621544338826,392.7330689342));
#49500=CARTESIAN_POINT('Ctrl Pts',(295.953168415807,-71.6325246163829,392.702345484388));
#49501=CARTESIAN_POINT('Ctrl Pts',(296.037660773368,-71.601797552647,392.67271616762));
#49502=CARTESIAN_POINT('Ctrl Pts',(296.052067301209,-71.5965583770343,392.667664165413));
#49503=CARTESIAN_POINT('Ctrl Pts',(296.066383106193,-71.591287185193,392.662643959429));
#49504=CARTESIAN_POINT('Ctrl Pts',(296.080609518588,-71.5859845479236,392.657655092465));
#49505=CARTESIAN_POINT('Ctrl Pts',(296.163364197678,-71.5551392417853,392.628634980214));
#49506=CARTESIAN_POINT('Ctrl Pts',(296.243092687893,-71.5232336033096,392.600675798085));
#49507=CARTESIAN_POINT('Ctrl Pts',(296.320007651119,-71.4903512772879,392.5737046794));
#49508=CARTESIAN_POINT('Ctrl Pts',(296.405578887035,-71.4537682619746,392.54369813889));
#49509=CARTESIAN_POINT('Ctrl Pts',(296.487669371849,-71.4159779683996,392.51490829633));
#49510=CARTESIAN_POINT('Ctrl Pts',(296.566499322963,-71.3770761149287,392.487264268723));
#49511=CARTESIAN_POINT('Ctrl Pts',(296.590594755396,-71.365185241364,392.47881450071));
#49512=CARTESIAN_POINT('Ctrl Pts',(296.614385651394,-71.3531901564309,392.470471746746));
#49513=CARTESIAN_POINT('Ctrl Pts',(296.637878473138,-71.341092656553,392.462233905615));
#49514=CARTESIAN_POINT('Ctrl Pts',(296.688139289384,-71.3152111245251,392.444609772429));
#49515=CARTESIAN_POINT('Ctrl Pts',(296.73703559184,-71.2888614634883,392.427465915853));
#49516=CARTESIAN_POINT('Ctrl Pts',(296.784610174726,-71.2620589084764,392.410788823981));
#49517=CARTESIAN_POINT('Ctrl Pts',(296.856519361253,-71.2215467313672,392.385581327932));
#49518=CARTESIAN_POINT('Ctrl Pts',(296.92542409753,-71.1799959836175,392.361421243769));
#49519=CARTESIAN_POINT('Ctrl Pts',(296.991253732561,-71.1375810950574,392.338337811185));
#49520=CARTESIAN_POINT('Ctrl Pts',(297.02886740447,-71.113346117884,392.325148422251));
#49521=CARTESIAN_POINT('Ctrl Pts',(297.065478074462,-71.088829010672,392.312310191884));
#49522=CARTESIAN_POINT('Ctrl Pts',(297.101079686947,-71.0640622089105,392.299825987935));
#49523=CARTESIAN_POINT('Ctrl Pts',(297.126698112609,-71.0462403624964,392.290842528241));
#49524=CARTESIAN_POINT('Ctrl Pts',(297.151794116107,-71.0282892411028,392.282042358285));
#49525=CARTESIAN_POINT('Ctrl Pts',(297.176362709175,-71.0102232726032,392.273427484222));
#49526=CARTESIAN_POINT('Ctrl Pts',(297.238139349407,-70.9647971941419,392.251765764558));
#49527=CARTESIAN_POINT('Ctrl Pts',(297.296594249163,-70.9186326263586,392.231273559932));
#49528=CARTESIAN_POINT('Ctrl Pts',(297.351737586078,-70.8719111276471,392.211942525523));
#49529=CARTESIAN_POINT('Ctrl Pts',(297.39400288267,-70.8361008537176,392.19712601371));
#49530=CARTESIAN_POINT('Ctrl Pts',(297.434323915126,-70.7999629729411,392.182991257644));
#49531=CARTESIAN_POINT('Ctrl Pts',(297.47272325268,-70.7635713397337,392.169528477904));
#49532=CARTESIAN_POINT('Ctrl Pts',(297.4802977877,-70.7563928382873,392.16687285145));
#49533=CARTESIAN_POINT('Ctrl Pts',(297.487797592225,-70.7492044430814,392.164243357357));
#49534=CARTESIAN_POINT('Ctrl Pts',(297.495222765696,-70.7420068815995,392.161639947474));
#49535=CARTESIAN_POINT('Ctrl Pts',(299.209414460475,-72.012007957416,391.000001627217));
#49536=CARTESIAN_POINT('Ctrl Pts',(299.163364790386,-71.9753249175646,391.000003616177));
#49537=CARTESIAN_POINT('Ctrl Pts',(299.116494777333,-71.9392458075241,391.002052727671));
#49538=CARTESIAN_POINT('Ctrl Pts',(299.069205430033,-71.9036114492888,391.006195158111));
#49539=CARTESIAN_POINT('Ctrl Pts',(299.022239451589,-71.8682207620344,391.010309262236));
#49540=CARTESIAN_POINT('Ctrl Pts',(298.974860013137,-71.8332687556906,391.016488185206));
#49541=CARTESIAN_POINT('Ctrl Pts',(298.927438390979,-71.7986331412756,391.024745193473));
#49542=CARTESIAN_POINT('Ctrl Pts',(298.88006471894,-71.7640325484769,391.03299385271));
#49543=CARTESIAN_POINT('Ctrl Pts',(298.832649141448,-71.7297478280264,391.043316415269));
#49544=CARTESIAN_POINT('Ctrl Pts',(298.785537542146,-71.6956899506139,391.055693654232));
#49545=CARTESIAN_POINT('Ctrl Pts',(298.759718399476,-71.6770247978908,391.062476903016));
#49546=CARTESIAN_POINT('Ctrl Pts',(298.733990114611,-71.6584283466725,391.069876702762));
#49547=CARTESIAN_POINT('Ctrl Pts',(298.708406203038,-71.6398898461304,391.077885749038));
#49548=CARTESIAN_POINT('Ctrl Pts',(298.641042885633,-71.5910773378212,391.098973842814));
#49549=CARTESIAN_POINT('Ctrl Pts',(298.574726333039,-71.5425836661342,391.124291348115));
#49550=CARTESIAN_POINT('Ctrl Pts',(298.509739437054,-71.4947553753244,391.153715969436));
#49551=CARTESIAN_POINT('Ctrl Pts',(298.446007898098,-71.4478509874047,391.182572193011));
#49552=CARTESIAN_POINT('Ctrl Pts',(298.383555320484,-71.4015866110902,391.215378436927));
#49553=CARTESIAN_POINT('Ctrl Pts',(298.322651474073,-71.3562721759616,391.25197246669));
#49554=CARTESIAN_POINT('Ctrl Pts',(298.292576717278,-71.3338955824275,391.270042861421));
#49555=CARTESIAN_POINT('Ctrl Pts',(298.262879642304,-71.3117503575619,391.289036158411));
#49556=CARTESIAN_POINT('Ctrl Pts',(298.233592745105,-71.2898721306231,391.308928412373));
#49557=CARTESIAN_POINT('Ctrl Pts',(298.179041925794,-71.2491209647858,391.345980434111));
#49558=CARTESIAN_POINT('Ctrl Pts',(298.125921199044,-71.2092859907837,391.386153790494));
#49559=CARTESIAN_POINT('Ctrl Pts',(298.074355627012,-71.1706830835568,391.429272972365));
#49560=CARTESIAN_POINT('Ctrl Pts',(298.022037552681,-71.131516839683,391.473021397396));
#49561=CARTESIAN_POINT('Ctrl Pts',(297.97132087597,-71.0936188702448,391.519802373784));
#49562=CARTESIAN_POINT('Ctrl Pts',(297.92234701012,-71.0572796433853,391.569397266211));
#49563=CARTESIAN_POINT('Ctrl Pts',(297.88768363514,-71.0315589814523,391.60450019965));
#49564=CARTESIAN_POINT('Ctrl Pts',(297.853893622557,-71.0066183661927,391.641012067787));
#49565=CARTESIAN_POINT('Ctrl Pts',(297.821027833467,-70.9825493079028,391.678844594721));
#49566=CARTESIAN_POINT('Ctrl Pts',(297.783852322583,-70.9553240513914,391.721638136449));
#49567=CARTESIAN_POINT('Ctrl Pts',(297.74783219056,-70.9292507855693,391.766122622644));
#49568=CARTESIAN_POINT('Ctrl Pts',(297.713249741123,-70.9041908400237,391.812136771624));
#49569=CARTESIAN_POINT('Ctrl Pts',(297.677888662821,-70.8785666661705,391.859186935841));
#49570=CARTESIAN_POINT('Ctrl Pts',(297.644030742679,-70.854002558325,391.907836549861));
#49571=CARTESIAN_POINT('Ctrl Pts',(297.611937753492,-70.8303782654378,391.957887372366));
#49572=CARTESIAN_POINT('Ctrl Pts',(297.578945979081,-70.8060923587238,392.009339901004));
#49573=CARTESIAN_POINT('Ctrl Pts',(297.547819508731,-70.7828005038815,392.062273279665));
#49574=CARTESIAN_POINT('Ctrl Pts',(297.518799775462,-70.760390068132,392.116443580042));
#49575=CARTESIAN_POINT('Ctrl Pts',(297.510781411271,-70.7541979011033,392.131411229564));
#49576=CARTESIAN_POINT('Ctrl Pts',(297.502923633929,-70.7480730855497,392.146473147346));
#49577=CARTESIAN_POINT('Ctrl Pts',(297.495230955743,-70.7420133331691,392.161623817083));
#49578=CARTESIAN_POINT('Origin',(293.564332522078,-74.552013924409,393.540000551893));
#49579=CARTESIAN_POINT('Origin',(297.262553908368,-69.47200726879,388.940612583843));
#49580=CARTESIAN_POINT('',(288.932479187181,-70.7420814892878,402.810893549063));
#49581=CARTESIAN_POINT('Origin',(287.218198108558,-69.47200726879,401.432533532013));
#49582=CARTESIAN_POINT('',(297.495223127598,-70.7420071496969,392.161640238453));
#49583=CARTESIAN_POINT('Origin',(287.218198108558,-69.47200726879,401.432533532013));
#49584=CARTESIAN_POINT('Origin',(287.218198108558,-69.47200726879,401.432533532013));
#49585=CARTESIAN_POINT('Origin',(287.218166972068,-69.4721721185271,401.432510673503));
#49586=CARTESIAN_POINT('Ctrl Pts',(291.203645131898,-69.4654484632099,403.635357625233));
#49587=CARTESIAN_POINT('Ctrl Pts',(291.173051143578,-69.4642529784631,403.617755948263));
#49588=CARTESIAN_POINT('Ctrl Pts',(290.972859048508,-69.461131317104,403.503668639343));
#49589=CARTESIAN_POINT('Ctrl Pts',(290.594946600108,-69.5121743079279,403.301685955943));
#49590=CARTESIAN_POINT('Ctrl Pts',(290.084964756368,-69.7115095210406,403.057939922303));
#49591=CARTESIAN_POINT('Ctrl Pts',(289.611953752488,-70.0335847626073,402.855968300073));
#49592=CARTESIAN_POINT('Ctrl Pts',(289.246049537548,-70.4242464530172,402.715633112443));
#49593=CARTESIAN_POINT('Ctrl Pts',(289.064520043938,-70.713413234504,402.651065852173));
#49594=CARTESIAN_POINT('Ctrl Pts',(288.998413612038,-70.840779768824,402.628068939403));
#49595=CARTESIAN_POINT('Ctrl Pts',(290.254313491288,-69.6040686220959,405.017443465873));
#49596=CARTESIAN_POINT('Ctrl Pts',(290.227163648548,-69.6012555491032,405.002376957633));
#49597=CARTESIAN_POINT('Ctrl Pts',(290.049137019188,-69.5867035136386,404.904544662123));
#49598=CARTESIAN_POINT('Ctrl Pts',(289.707639443108,-69.605895880883,404.728653457343));
#49599=CARTESIAN_POINT('Ctrl Pts',(289.225829971688,-69.7468138148854,404.504512583233));
#49600=CARTESIAN_POINT('Ctrl Pts',(288.753707550808,-70.0122251216757,404.303173476413));
#49601=CARTESIAN_POINT('Ctrl Pts',(288.366767689408,-70.3697189200571,404.149170983363));
#49602=CARTESIAN_POINT('Ctrl Pts',(288.166452102968,-70.653842506004,404.072518279053));
#49603=CARTESIAN_POINT('Ctrl Pts',(288.092556015588,-70.781931585494,404.044593288783));
#49604=CARTESIAN_POINT('Ctrl Pts',(289.621245193278,-68.419135189814,406.030249678763));
#49605=CARTESIAN_POINT('Ctrl Pts',(289.582956330878,-68.41446975451,406.006060540213));
#49606=CARTESIAN_POINT('Ctrl Pts',(289.332024190148,-68.389529900869,405.848495325453));
#49607=CARTESIAN_POINT('Ctrl Pts',(288.852027174878,-68.410079767087,405.558979345753));
#49608=CARTESIAN_POINT('Ctrl Pts',(288.174342656098,-68.6071111008892,405.175179965833));
#49609=CARTESIAN_POINT('Ctrl Pts',(287.507154848008,-68.9922445608695,404.816936851443));
#49610=CARTESIAN_POINT('Ctrl Pts',(286.956624676828,-69.522348198985,404.533699690253));
#49611=CARTESIAN_POINT('Ctrl Pts',(286.670012222648,-69.9492631288261,404.389800539313));
#49612=CARTESIAN_POINT('Ctrl Pts',(286.564094264238,-70.1425137073577,404.337074995393));
#49613=CARTESIAN_POINT('Ctrl Pts',(289.749096409928,-66.742924819268,405.962398778943));
#49614=CARTESIAN_POINT('Ctrl Pts',(289.692909216458,-66.737473314687,405.923836788043));
#49615=CARTESIAN_POINT('Ctrl Pts',(289.325208151628,-66.710484421782,405.672506085923));
#49616=CARTESIAN_POINT('Ctrl Pts',(288.629076985118,-66.764646425836,405.209457145263));
#49617=CARTESIAN_POINT('Ctrl Pts',(287.669049228958,-67.092908761381,404.598876954383));
#49618=CARTESIAN_POINT('Ctrl Pts',(286.747852601878,-67.690059702462,404.036399957943));
#49619=CARTESIAN_POINT('Ctrl Pts',(286.006080448558,-68.4773127599906,403.599132951133));
#49620=CARTESIAN_POINT('Ctrl Pts',(285.626273772118,-69.0945594144157,403.380059086583));
#49621=CARTESIAN_POINT('Ctrl Pts',(285.486593332898,-69.3716421412076,403.300079990813));
#49622=CARTESIAN_POINT('Ctrl Pts',(290.999733508293,-69.4720072796082,403.750310918259));
#49623=CARTESIAN_POINT('Ctrl Pts',(290.872577534336,-69.472005849716,403.678659148785));
#49624=CARTESIAN_POINT('Ctrl Pts',(290.743479119672,-69.4843168520742,403.608952691824));
#49625=CARTESIAN_POINT('Ctrl Pts',(290.573417073416,-69.5166114182824,403.52069155269));
#49626=CARTESIAN_POINT('Ctrl Pts',(290.532260427764,-69.5256727717997,403.499602683094));
#49627=CARTESIAN_POINT('Ctrl Pts',(290.403656894431,-69.5579244915856,403.434557401163));
#49628=CARTESIAN_POINT('Ctrl Pts',(290.316431600513,-69.5855055086998,403.391675607924));
#49629=CARTESIAN_POINT('Ctrl Pts',(290.149149606719,-69.6496600928294,403.311655708688));
#49630=CARTESIAN_POINT('Ctrl Pts',(290.069003164979,-69.6855216028275,403.274325295143));
#49631=CARTESIAN_POINT('Ctrl Pts',(289.944724104076,-69.7495837444736,403.217895622591));
#49632=CARTESIAN_POINT('Ctrl Pts',(289.899775287176,-69.7745536342543,403.197796416373));
#49633=CARTESIAN_POINT('Ctrl Pts',(289.739386970048,-69.8703147051977,403.127097475838));
#49634=CARTESIAN_POINT('Ctrl Pts',(289.62693747088,-69.950164289824,403.079509070807));
#49635=CARTESIAN_POINT('Ctrl Pts',(289.514831043793,-70.0443954690097,403.033665288188));
#49636=CARTESIAN_POINT('Ctrl Pts',(289.509507836765,-70.0489065579999,403.031492461485));
#49637=CARTESIAN_POINT('Ctrl Pts',(289.392695719642,-70.1487082562832,402.983898553237));
#49638=CARTESIAN_POINT('Ctrl Pts',(289.287584575188,-70.2548440769942,402.942824966919));
#49639=CARTESIAN_POINT('Ctrl Pts',(289.16570429737,-70.4011757050269,402.896533092463));
#49640=CARTESIAN_POINT('Ctrl Pts',(289.140508058321,-70.4328767762964,402.887047510866));
#49641=CARTESIAN_POINT('Ctrl Pts',(289.049504035329,-70.5529932331026,402.853066472181));
#49642=CARTESIAN_POINT('Ctrl Pts',(288.988121244777,-70.6454659295424,402.830716147373));
#49643=CARTESIAN_POINT('Ctrl Pts',(288.932529004827,-70.7420200540542,402.810888197655));
#49644=CARTESIAN_POINT('Origin',(290.999736346768,-66.932007290493,403.750312537073));
#49645=CARTESIAN_POINT('Origin',(301.593507745258,-72.01200726879,390.575096505143));
#49646=CARTESIAN_POINT('Origin',(299.209522825618,-72.01200726879,393.540000551893));
#49647=CARTESIAN_POINT('Origin',(299.209522825618,-72.01200726879,393.540000551893));
#49648=CARTESIAN_POINT('Origin',(299.209522825618,-72.01200726879,393.540000551893));
#49649=CARTESIAN_POINT('Origin',(220.367523674428,-72.0120072687899,393.540000551893));
#49650=CARTESIAN_POINT('Origin',(263.115917770968,-66.93200726879,445.000000551893));
#49651=CARTESIAN_POINT('Origin',(304.365605883138,-66.93200726879,417.116182114513));
#49652=CARTESIAN_POINT('Ctrl Pts',(305.487892930988,-70.84102555105,419.117632653513));
#49653=CARTESIAN_POINT('Ctrl Pts',(305.464850568738,-70.713370333766,419.051393351193));
#49654=CARTESIAN_POINT('Ctrl Pts',(305.400366416118,-70.4246254735271,418.870097571243));
#49655=CARTESIAN_POINT('Ctrl Pts',(305.260591345888,-70.03536275261,418.505648539213));
#49656=CARTESIAN_POINT('Ctrl Pts',(305.059765698908,-69.713847880508,418.035004394313));
#49657=CARTESIAN_POINT('Ctrl Pts',(304.816679242508,-69.5133172296705,417.525769821493));
#49658=CARTESIAN_POINT('Ctrl Pts',(304.613886321128,-69.461221631883,417.145987521843));
#49659=CARTESIAN_POINT('Ctrl Pts',(304.498796499068,-69.4642140921142,416.943973415093));
#49660=CARTESIAN_POINT('Ctrl Pts',(304.480695707958,-69.4654397984238,416.912510521983));
#49661=CARTESIAN_POINT('Ctrl Pts',(304.071378819998,-70.782178593213,420.023505505583));
#49662=CARTESIAN_POINT('Ctrl Pts',(304.043397780898,-70.653795640172,419.949459441043));
#49663=CARTESIAN_POINT('Ctrl Pts',(303.966843753868,-70.3700937613876,419.749402599143));
#49664=CARTESIAN_POINT('Ctrl Pts',(303.813452007048,-70.0138432466799,419.363994547833));
#49665=CARTESIAN_POINT('Ctrl Pts',(303.613137828218,-69.7486471121801,418.894056400303));
#49666=CARTESIAN_POINT('Ctrl Pts',(303.389433232488,-69.6065541583208,418.412681539603));
#49667=CARTESIAN_POINT('Ctrl Pts',(303.212782003088,-69.5866015108646,418.069396475333));
#49668=CARTESIAN_POINT('Ctrl Pts',(303.114084903818,-69.6011568594992,417.889736153403));
#49669=CARTESIAN_POINT('Ctrl Pts',(303.098591120058,-69.604046788924,417.861814842233));
#49670=CARTESIAN_POINT('Ctrl Pts',(303.778945393968,-70.1428866111332,421.552028656883));
#49671=CARTESIAN_POINT('Ctrl Pts',(303.726113566768,-69.9491917586301,421.445895462313));
#49672=CARTESIAN_POINT('Ctrl Pts',(303.582399730018,-69.5229124456986,421.159653521583));
#49673=CARTESIAN_POINT('Ctrl Pts',(303.300284792268,-68.9946418506595,420.611300963493));
#49674=CARTESIAN_POINT('Ctrl Pts',(302.943787010338,-68.6097419549074,419.947170649373));
#49675=CARTESIAN_POINT('Ctrl Pts',(302.560567407998,-68.410944976237,419.270074416423));
#49676=CARTESIAN_POINT('Ctrl Pts',(302.269706171108,-68.389326074635,418.787576198633));
#49677=CARTESIAN_POINT('Ctrl Pts',(302.110731762418,-68.414305770954,418.534345416843));
#49678=CARTESIAN_POINT('Ctrl Pts',(302.085856285908,-68.419099312278,418.494968636633));
#49679=CARTESIAN_POINT('Ctrl Pts',(304.815992739688,-69.3721770309352,422.629594373163));
#49680=CARTESIAN_POINT('Ctrl Pts',(304.735852768918,-69.0944600428793,422.489631115633));
#49681=CARTESIAN_POINT('Ctrl Pts',(304.517061054368,-68.4781267582278,422.110314934323));
#49682=CARTESIAN_POINT('Ctrl Pts',(304.081529312988,-67.693627670349,421.371481733023));
#49683=CARTESIAN_POINT('Ctrl Pts',(303.521853468128,-67.097079327632,420.454658245163));
#49684=CARTESIAN_POINT('Ctrl Pts',(302.912262522438,-66.766264510463,419.495730799533));
#49685=CARTESIAN_POINT('Ctrl Pts',(302.447058675868,-66.710340497794,418.796089905903));
#49686=CARTESIAN_POINT('Ctrl Pts',(302.193474645818,-66.737284122907,418.425039014543));
#49687=CARTESIAN_POINT('Ctrl Pts',(302.153818312178,-66.742883601451,418.367255833933));
#49688=CARTESIAN_POINT('',(305.30504375147,-70.7420553610057,419.183412677393));
#49689=CARTESIAN_POINT('Origin',(306.683409048718,-69.4721778291691,420.897753867533));
#49690=CARTESIAN_POINT('Ctrl Pts',(305.305042220708,-70.742010897001,419.183399964073));
#49691=CARTESIAN_POINT('Ctrl Pts',(305.277815995278,-70.609423932929,419.107063253613));
#49692=CARTESIAN_POINT('Ctrl Pts',(305.213936898318,-70.3602758137963,418.932833631543));
#49693=CARTESIAN_POINT('Ctrl Pts',(305.091118039558,-70.0432002664174,418.618591900583));
#49694=CARTESIAN_POINT('Ctrl Pts',(304.942919608568,-69.791339768846,418.267516581863));
#49695=CARTESIAN_POINT('Ctrl Pts',(304.771191547518,-69.6083606197754,417.892354850793));
#49696=CARTESIAN_POINT('Ctrl Pts',(304.578280667416,-69.4970261598067,417.504572957698));
#49697=CARTESIAN_POINT('Ctrl Pts',(304.437924443537,-69.4720061889132,417.244522589505));
#49698=CARTESIAN_POINT('Ctrl Pts',(304.365607433868,-69.4720072829599,417.116184866493));
#49699=CARTESIAN_POINT('Origin',(208.730420887858,-72.01200726879,494.013388642063));
#49700=CARTESIAN_POINT('',(315.954292413807,-70.7420026857022,410.620680697854));
#49701=CARTESIAN_POINT('',(305.305042220708,-70.742010897001,419.183399964073));
#49702=CARTESIAN_POINT('Origin',(314.575917770968,-72.01200726879,408.906395497243));
#49703=CARTESIAN_POINT('Origin',(314.575917770968,-72.01200726879,408.906395497243));
#49704=CARTESIAN_POINT('Origin',(314.575917770968,-72.011994055132,408.906387830823));
#49705=CARTESIAN_POINT('Ctrl Pts',(316.576327554178,-72.767751257,407.522814320583));
#49706=CARTESIAN_POINT('Ctrl Pts',(316.583782922478,-72.841526713075,407.585316356403));
#49707=CARTESIAN_POINT('Ctrl Pts',(316.619560336498,-73.179288192142,407.887183345043));
#49708=CARTESIAN_POINT('Ctrl Pts',(316.689891498608,-73.717781820139,408.502271310003));
#49709=CARTESIAN_POINT('Ctrl Pts',(316.787434179168,-74.277385903423,409.428236779663));
#49710=CARTESIAN_POINT('Ctrl Pts',(316.886554255398,-74.694184456929,410.486632004843));
#49711=CARTESIAN_POINT('Ctrl Pts',(316.980630255158,-74.948821569849,411.678956305813));
#49712=CARTESIAN_POINT('Ctrl Pts',(317.060241543218,-75.007840422917,412.999175337793));
#49713=CARTESIAN_POINT('Ctrl Pts',(317.097721793168,-74.879327723335,414.019184250283));
#49714=CARTESIAN_POINT('Ctrl Pts',(317.108843213778,-74.744596630044,414.592201564763));
#49715=CARTESIAN_POINT('Ctrl Pts',(317.110701299278,-74.713685427546,414.711610886703));
#49716=CARTESIAN_POINT('Ctrl Pts',(317.613103449168,-72.015040141213,408.613288514213));
#49717=CARTESIAN_POINT('Ctrl Pts',(317.614247001878,-72.069657434211,408.668567963553));
#49718=CARTESIAN_POINT('Ctrl Pts',(317.619313854468,-72.318399048559,408.935215997553));
#49719=CARTESIAN_POINT('Ctrl Pts',(317.624814914728,-72.703469476734,409.475218706333));
#49720=CARTESIAN_POINT('Ctrl Pts',(317.618445020368,-73.078553800105,410.278931984853));
#49721=CARTESIAN_POINT('Ctrl Pts',(317.590746058588,-73.326904151249,411.185995219963));
#49722=CARTESIAN_POINT('Ctrl Pts',(317.531896134968,-73.435351582353,412.193514319393));
#49723=CARTESIAN_POINT('Ctrl Pts',(317.429510279318,-73.381806590394,413.291266192613));
#49724=CARTESIAN_POINT('Ctrl Pts',(317.314886825698,-73.209045637398,414.123357625123));
#49725=CARTESIAN_POINT('Ctrl Pts',(317.235911832778,-73.066698954042,414.584338071243));
#49726=CARTESIAN_POINT('Ctrl Pts',(317.218779455948,-73.035006784976,414.680100276573));
#49727=CARTESIAN_POINT('Ctrl Pts',(317.277494481808,-71.078506845443,409.970079907573));
#49728=CARTESIAN_POINT('Ctrl Pts',(317.270785073228,-71.113684992587,410.009998731183));
#49729=CARTESIAN_POINT('Ctrl Pts',(317.237893413858,-71.274294562834,410.202906766823));
#49730=CARTESIAN_POINT('Ctrl Pts',(317.165882438868,-71.526452514999,410.597081606803));
#49731=CARTESIAN_POINT('Ctrl Pts',(317.042927735698,-71.779984116282,411.193539961963));
#49732=CARTESIAN_POINT('Ctrl Pts',(316.882986923958,-71.958291490743,411.879151906023));
#49733=CARTESIAN_POINT('Ctrl Pts',(316.677499107228,-72.052539059859,412.656275961963));
#49734=CARTESIAN_POINT('Ctrl Pts',(316.416904371818,-72.047682890276,413.522680104983));
#49735=CARTESIAN_POINT('Ctrl Pts',(316.184702855868,-71.960063670979,414.197393038243));
#49736=CARTESIAN_POINT('Ctrl Pts',(316.041666670348,-71.881362788512,414.578578626823));
#49737=CARTESIAN_POINT('Ctrl Pts',(316.011276520298,-71.863634441064,414.658112344523));
#49738=CARTESIAN_POINT('Ctrl Pts',(315.805224721488,-70.615950955131,410.640209231163));
#49739=CARTESIAN_POINT('Ctrl Pts',(315.794636946478,-70.645062585471,410.667418342263));
#49740=CARTESIAN_POINT('Ctrl Pts',(315.743200015988,-70.780329866031,410.799858625583));
#49741=CARTESIAN_POINT('Ctrl Pts',(315.635437754638,-71.013440751854,411.079889146753));
#49742=CARTESIAN_POINT('Ctrl Pts',(315.465112514288,-71.293762523166,411.529660968353));
#49743=CARTESIAN_POINT('Ctrl Pts',(315.260390694088,-71.549628732834,412.079244646643));
#49744=CARTESIAN_POINT('Ctrl Pts',(315.017548119678,-71.771639918357,412.742208030733));
#49745=CARTESIAN_POINT('Ctrl Pts',(314.733655070238,-71.942527322346,413.530877231093));
#49746=CARTESIAN_POINT('Ctrl Pts',(314.500985277318,-72.009638215756,414.189289707313));
#49747=CARTESIAN_POINT('Ctrl Pts',(314.364918237878,-72.021141169012,414.578968533643));
#49748=CARTESIAN_POINT('Ctrl Pts',(314.336314960658,-72.022313562161,414.661090911573));
#49749=CARTESIAN_POINT('Ctrl Pts',(315.954278372765,-70.7420068809478,410.620695559264));
#49750=CARTESIAN_POINT('Ctrl Pts',(315.951674963195,-70.7492044424186,410.628120732305));
#49751=CARTESIAN_POINT('Ctrl Pts',(315.949045469402,-70.7563928376237,410.635620536423));
#49752=CARTESIAN_POINT('Ctrl Pts',(315.946389843238,-70.7635713390688,410.643195071058));
#49753=CARTESIAN_POINT('Ctrl Pts',(315.928825029924,-70.8110513042364,410.693294474588));
#49754=CARTESIAN_POINT('Ctrl Pts',(315.910115871374,-70.8580999963981,410.746666500798));
#49755=CARTESIAN_POINT('Ctrl Pts',(315.890242304815,-70.9045511124985,410.803356320062));
#49756=CARTESIAN_POINT('Ctrl Pts',(315.875009939518,-70.9401542019987,410.846807002811));
#49757=CARTESIAN_POINT('Ctrl Pts',(315.85909374957,-70.975405861412,410.892206097532));
#49758=CARTESIAN_POINT('Ctrl Pts',(315.842490840838,-71.0102232739626,410.939555612702));
#49759=CARTESIAN_POINT('Ctrl Pts',(315.833875966783,-71.0282892423347,410.964124205851));
#49760=CARTESIAN_POINT('Ctrl Pts',(315.825075796751,-71.0462403635193,410.98922020942));
#49761=CARTESIAN_POINT('Ctrl Pts',(315.816092336927,-71.0640622097132,411.014838635134));
#49762=CARTESIAN_POINT('Ctrl Pts',(315.794243070786,-71.1074078992631,411.077146900826));
#49763=CARTESIAN_POINT('Ctrl Pts',(315.771308437755,-71.1499888075381,411.142548617801));
#49764=CARTESIAN_POINT('Ctrl Pts',(315.747307516489,-71.1916308944392,411.211001129355));
#49765=CARTESIAN_POINT('Ctrl Pts',(315.733593917851,-71.2154242671948,411.250113389202));
#49766=CARTESIAN_POINT('Ctrl Pts',(315.719532516711,-71.2389111258158,411.290220793764));
#49767=CARTESIAN_POINT('Ctrl Pts',(315.705129498392,-71.2620589077046,411.331308147898));
#49768=CARTESIAN_POINT('Ctrl Pts',(315.688452406246,-71.2888614627661,411.378882730932));
#49769=CARTESIAN_POINT('Ctrl Pts',(315.671308549575,-71.3152111239888,411.427779033538));
#49770=CARTESIAN_POINT('Ctrl Pts',(315.653684416389,-71.3410926562256,411.478039849955));
#49771=CARTESIAN_POINT('Ctrl Pts',(315.626733718716,-71.3806705091198,411.554898328823));
#49772=CARTESIAN_POINT('Ctrl Pts',(315.598659847284,-71.4191559802297,411.634947740602));
#49773=CARTESIAN_POINT('Ctrl Pts',(315.569390399603,-71.4564687983853,411.718411883613));
#49774=CARTESIAN_POINT('Ctrl Pts',(315.560443806303,-71.4678739541145,411.743923801391));
#49775=CARTESIAN_POINT('Ctrl Pts',(315.551385540596,-71.4791691936542,411.769754688635));
#49776=CARTESIAN_POINT('Ctrl Pts',(315.54221364373,-71.4903512773119,411.795910671373));
#49777=CARTESIAN_POINT('Ctrl Pts',(315.515242525184,-71.5232336034354,411.8728256347));
#49778=CARTESIAN_POINT('Ctrl Pts',(315.487283343028,-71.5551392419007,411.952554125022));
#49779=CARTESIAN_POINT('Ctrl Pts',(315.458263230685,-71.5859845480198,412.035308804217));
#49780=CARTESIAN_POINT('Ctrl Pts',(315.429004195628,-71.6170838036807,412.118744803052));
#49781=CARTESIAN_POINT('Ctrl Pts',(315.398666821627,-71.6471054203413,412.205256651372));
#49782=CARTESIAN_POINT('Ctrl Pts',(315.367160717853,-71.6759139021885,412.295107683839));
#49783=CARTESIAN_POINT('Ctrl Pts',(315.361788708047,-71.6808259486952,412.310427909753));
#49784=CARTESIAN_POINT('Ctrl Pts',(315.356382733281,-71.6857026097516,412.325845178458));
#49785=CARTESIAN_POINT('Ctrl Pts',(315.350942364032,-71.6905430691911,412.341360743912));
#49786=CARTESIAN_POINT('Ctrl Pts',(315.320097573025,-71.7179866034364,412.429328003468));
#49787=CARTESIAN_POINT('Ctrl Pts',(315.288149145133,-71.7442659054153,412.520446812886));
#49788=CARTESIAN_POINT('Ctrl Pts',(315.255030549156,-71.769198804243,412.614896704636));
#49789=CARTESIAN_POINT('Ctrl Pts',(315.244780981062,-71.7769150566009,412.644127128461));
#49790=CARTESIAN_POINT('Ctrl Pts',(315.234419413948,-71.7845020756706,412.673676369388));
#49791=CARTESIAN_POINT('Ctrl Pts',(315.223944109765,-71.7919537134942,412.703549064507));
#49792=CARTESIAN_POINT('Ctrl Pts',(315.192555945547,-71.814281774581,412.793059501975));
#49793=CARTESIAN_POINT('Ctrl Pts',(315.160146055062,-71.8353967743902,412.88547564147));
#49794=CARTESIAN_POINT('Ctrl Pts',(315.126657947258,-71.855100815038,412.980949644988));
#49795=CARTESIAN_POINT('Ctrl Pts',(315.093751173053,-71.874462805279,413.074766276684));
#49796=CARTESIAN_POINT('Ctrl Pts',(315.059816408482,-71.8924577821927,413.171525236941));
#49797=CARTESIAN_POINT('Ctrl Pts',(315.024927819642,-71.9088265655513,413.271013891659));
#49798=CARTESIAN_POINT('Ctrl Pts',(314.998821176152,-71.9210750973982,413.345459861713));
#49799=CARTESIAN_POINT('Ctrl Pts',(314.972180772578,-71.9324134528439,413.421433367158));
#49800=CARTESIAN_POINT('Ctrl Pts',(314.945043412244,-71.9427410029756,413.498828889789));
#49801=CARTESIAN_POINT('Ctrl Pts',(314.919424047628,-71.9524908559149,413.571895101447));
#49802=CARTESIAN_POINT('Ctrl Pts',(314.89336186585,-71.9613399669071,413.64622841268));
#49803=CARTESIAN_POINT('Ctrl Pts',(314.86688749706,-71.9692011295698,413.721740936061));
#49804=CARTESIAN_POINT('Ctrl Pts',(314.828142974388,-71.980705728506,413.832251471643));
#49805=CARTESIAN_POINT('Ctrl Pts',(314.788516830115,-71.99009665066,413.945279068244));
#49806=CARTESIAN_POINT('Ctrl Pts',(314.748000519617,-71.9971271824969,414.060838741406));
#49807=CARTESIAN_POINT('Ctrl Pts',(314.70748420912,-72.0041577143339,414.176398414569));
#49808=CARTESIAN_POINT('Ctrl Pts',(314.666077513173,-72.0088279534613,414.294490762271));
#49809=CARTESIAN_POINT('Ctrl Pts',(314.623786099889,-72.0108586572646,414.415090195384));
#49810=CARTESIAN_POINT('Ctrl Pts',(314.607953565646,-72.0116188869426,414.460238713869));
#49811=CARTESIAN_POINT('Ctrl Pts',(314.591997198208,-72.012008864435,414.505738145661));
#49812=CARTESIAN_POINT('Ctrl Pts',(314.575917770983,-72.0120105964115,414.551585801107));
#49813=CARTESIAN_POINT('Origin',(314.575917770968,-74.55200726879,414.551585801123));
#49814=CARTESIAN_POINT('Origin',(314.575917770968,-74.55200726879,402.251606455353));
#49815=CARTESIAN_POINT('Origin',(314.575917770968,-74.5520139244091,475.448415303003));
#49816=CARTESIAN_POINT('Ctrl Pts',(317.110711991638,-74.7135074441071,475.287702781083));
#49817=CARTESIAN_POINT('Ctrl Pts',(317.108852221438,-74.7444877320721,475.407336443503));
#49818=CARTESIAN_POINT('Ctrl Pts',(317.097730648738,-74.879297233076,475.980574777393));
#49819=CARTESIAN_POINT('Ctrl Pts',(317.060241556308,-75.0078404229241,477.000825766993));
#49820=CARTESIAN_POINT('Ctrl Pts',(316.980630251068,-74.9488215722141,478.321044798713));
#49821=CARTESIAN_POINT('Ctrl Pts',(316.886554256118,-74.6941844595181,479.513369099403));
#49822=CARTESIAN_POINT('Ctrl Pts',(316.787434174568,-74.2773859025651,480.571764327013));
#49823=CARTESIAN_POINT('Ctrl Pts',(316.689891508138,-73.7177818299221,481.497729789503));
#49824=CARTESIAN_POINT('Ctrl Pts',(316.619540328858,-73.1791351904631,482.112992516613));
#49825=CARTESIAN_POINT('Ctrl Pts',(316.583745197778,-72.8411704404731,482.415003143143));
#49826=CARTESIAN_POINT('Ctrl Pts',(316.576271949218,-72.7672009368351,482.477652958003));
#49827=CARTESIAN_POINT('Ctrl Pts',(317.218680820108,-73.034824311939,475.319349530363));
#49828=CARTESIAN_POINT('Ctrl Pts',(317.235848029108,-73.066583901593,475.415290483253));
#49829=CARTESIAN_POINT('Ctrl Pts',(317.314859582928,-73.209004644328,475.876445999973));
#49830=CARTESIAN_POINT('Ctrl Pts',(317.429510295178,-73.3818065881171,476.708734911823));
#49831=CARTESIAN_POINT('Ctrl Pts',(317.531896132978,-73.435351583061,477.806486784543));
#49832=CARTESIAN_POINT('Ctrl Pts',(317.590746061838,-73.3269041523451,478.814005883533));
#49833=CARTESIAN_POINT('Ctrl Pts',(317.618445018148,-73.0785537983271,479.721069121113));
#49834=CARTESIAN_POINT('Ctrl Pts',(317.624814927498,-72.7034694849991,480.524782392033));
#49835=CARTESIAN_POINT('Ctrl Pts',(317.619312266038,-72.3182896344501,481.064938532713));
#49836=CARTESIAN_POINT('Ctrl Pts',(317.614241673058,-72.0693950602571,481.331714387203));
#49837=CARTESIAN_POINT('Ctrl Pts',(317.613094923088,-72.0146327241461,481.387124895043));
#49838=CARTESIAN_POINT('Ctrl Pts',(316.011101558728,-71.8635323633291,475.341430884903));
#49839=CARTESIAN_POINT('Ctrl Pts',(316.041551082658,-71.8812991757081,475.421114413693));
#49840=CARTESIAN_POINT('Ctrl Pts',(316.184647725488,-71.9600428790521,475.802447937593));
#49841=CARTESIAN_POINT('Ctrl Pts',(316.416904379748,-72.0476828872321,476.477320998843));
#49842=CARTESIAN_POINT('Ctrl Pts',(316.677499105488,-72.0525390584191,477.343725141293));
#49843=CARTESIAN_POINT('Ctrl Pts',(316.882986925318,-71.9582914896151,478.120849196703));
#49844=CARTESIAN_POINT('Ctrl Pts',(317.042927734188,-71.7799841135891,478.806461141873));
#49845=CARTESIAN_POINT('Ctrl Pts',(317.165882445818,-71.5264525183511,479.402919492593));
#49846=CARTESIAN_POINT('Ctrl Pts',(317.237913857528,-71.2742229144981,479.797206326403));
#49847=CARTESIAN_POINT('Ctrl Pts',(317.270819774818,-71.1135155794621,479.990205841383));
#49848=CARTESIAN_POINT('Ctrl Pts',(317.277544524948,-71.0782444347641,480.030218930233));
#49849=CARTESIAN_POINT('Ctrl Pts',(314.336150287048,-72.0223202985271,475.338437405843));
#49850=CARTESIAN_POINT('Ctrl Pts',(314.364808267128,-72.0211504616851,475.420717639173));
#49851=CARTESIAN_POINT('Ctrl Pts',(314.500930059328,-72.009654141941,475.810555138393));
#49852=CARTESIAN_POINT('Ctrl Pts',(314.733655066588,-71.9425273225521,476.469123872633));
#49853=CARTESIAN_POINT('Ctrl Pts',(315.017548117408,-71.7716399178201,477.257793072913));
#49854=CARTESIAN_POINT('Ctrl Pts',(315.260390691488,-71.549628732325,477.920756456873));
#49855=CARTESIAN_POINT('Ctrl Pts',(315.465112512148,-71.2937625221141,478.470340134773));
#49856=CARTESIAN_POINT('Ctrl Pts',(315.635437751448,-71.0134407520801,478.920111956783));
#49857=CARTESIAN_POINT('Ctrl Pts',(315.743230630368,-70.7802636373911,479.200222031243));
#49858=CARTESIAN_POINT('Ctrl Pts',(315.794691197048,-70.6449199031991,479.332722454313));
#49859=CARTESIAN_POINT('Ctrl Pts',(315.805303686998,-70.6157338063321,479.359994807443));
#49860=CARTESIAN_POINT('',(315.954294408643,-70.7420091884829,479.37931719287));
#49861=CARTESIAN_POINT('Ctrl Pts',(314.575917770969,-72.0120105965992,475.448415302637));
#49862=CARTESIAN_POINT('Ctrl Pts',(314.591997198235,-72.012008864552,475.494262958081));
#49863=CARTESIAN_POINT('Ctrl Pts',(314.607953565725,-72.0116188869949,475.539762389914));
#49864=CARTESIAN_POINT('Ctrl Pts',(314.6237861,-72.0108586572668,475.5849109084));
#49865=CARTESIAN_POINT('Ctrl Pts',(314.66607751335,-72.0088279533304,475.70551034146));
#49866=CARTESIAN_POINT('Ctrl Pts',(314.70748420933,-72.0041577141727,475.823602689117));
#49867=CARTESIAN_POINT('Ctrl Pts',(314.748000519834,-71.997127182348,475.939162362245));
#49868=CARTESIAN_POINT('Ctrl Pts',(314.788516830339,-71.9900966505232,476.054722035374));
#49869=CARTESIAN_POINT('Ctrl Pts',(314.828142974591,-71.9807057284241,476.167749631951));
#49870=CARTESIAN_POINT('Ctrl Pts',(314.866887497221,-71.969201129537,476.27826016752));
#49871=CARTESIAN_POINT('Ctrl Pts',(314.89336186601,-71.9613399668997,476.353772690968));
#49872=CARTESIAN_POINT('Ctrl Pts',(314.919424047776,-71.9524908559287,476.428106002271));
#49873=CARTESIAN_POINT('Ctrl Pts',(314.945043412379,-71.9427410029957,476.501172213995));
#49874=CARTESIAN_POINT('Ctrl Pts',(314.981309437727,-71.9289393955363,476.604602612351));
#49875=CARTESIAN_POINT('Ctrl Pts',(315.016687357102,-71.9133317336536,476.705491735856));
#49876=CARTESIAN_POINT('Ctrl Pts',(315.051091306944,-71.8961610227584,476.803593407501));
#49877=CARTESIAN_POINT('Ctrl Pts',(315.076835302516,-71.8833124194068,476.877001519419));
#49878=CARTESIAN_POINT('Ctrl Pts',(315.102034267479,-71.8695891220288,476.948849783074));
#49879=CARTESIAN_POINT('Ctrl Pts',(315.12665794713,-71.8551008150864,477.019051458575));
#49880=CARTESIAN_POINT('Ctrl Pts',(315.160146054969,-71.8353967744164,477.114525462175));
#49881=CARTESIAN_POINT('Ctrl Pts',(315.192555945518,-71.8142817745934,477.206941601741));
#49882=CARTESIAN_POINT('Ctrl Pts',(315.223944109793,-71.7919537135017,477.296452039276));
#49883=CARTESIAN_POINT('Ctrl Pts',(315.25779210891,-71.7678758418075,477.39297725127));
#49884=CARTESIAN_POINT('Ctrl Pts',(315.290451662713,-71.742387394248,477.486122598949));
#49885=CARTESIAN_POINT('Ctrl Pts',(315.32198579055,-71.715682443271,477.576057318069));
#49886=CARTESIAN_POINT('Ctrl Pts',(315.33174499568,-71.7074177753551,477.603890381244));
#49887=CARTESIAN_POINT('Ctrl Pts',(315.34139649519,-71.6990363146508,477.631416186877));
#49888=CARTESIAN_POINT('Ctrl Pts',(315.350942363955,-71.690543069327,477.658640359569));
#49889=CARTESIAN_POINT('Ctrl Pts',(315.382849388659,-71.6621544338846,477.749637038026));
#49890=CARTESIAN_POINT('Ctrl Pts',(315.413572838469,-71.6325246163871,477.83725119672));
#49891=CARTESIAN_POINT('Ctrl Pts',(315.443202155235,-71.6017975526535,477.921743554275));
#49892=CARTESIAN_POINT('Ctrl Pts',(315.448254157444,-71.5965583770387,477.936150082122));
#49893=CARTESIAN_POINT('Ctrl Pts',(315.453274363431,-71.5912871851952,477.950465887112));
#49894=CARTESIAN_POINT('Ctrl Pts',(315.458263230396,-71.5859845479237,477.964692299512));
#49895=CARTESIAN_POINT('Ctrl Pts',(315.487283342647,-71.5551392417853,478.047446978603));
#49896=CARTESIAN_POINT('Ctrl Pts',(315.515242524777,-71.5232336033097,478.127175468818));
#49897=CARTESIAN_POINT('Ctrl Pts',(315.542213643461,-71.4903512772878,478.204090432044));
#49898=CARTESIAN_POINT('Ctrl Pts',(315.572220183972,-71.4537682619738,478.289661667962));
#49899=CARTESIAN_POINT('Ctrl Pts',(315.601010026533,-71.4159779683979,478.371752152777));
#49900=CARTESIAN_POINT('Ctrl Pts',(315.62865405414,-71.3770761149262,478.450582103894));
#49901=CARTESIAN_POINT('Ctrl Pts',(315.637103822152,-71.3651852413623,478.474677536325));
#49902=CARTESIAN_POINT('Ctrl Pts',(315.645446576115,-71.3531901564301,478.498468432321));
#49903=CARTESIAN_POINT('Ctrl Pts',(315.653684417246,-71.341092656553,478.521961254064));
#49904=CARTESIAN_POINT('Ctrl Pts',(315.671308550432,-71.3152111245253,478.572222070309));
#49905=CARTESIAN_POINT('Ctrl Pts',(315.688452407008,-71.2888614634885,478.621118372765));
#49906=CARTESIAN_POINT('Ctrl Pts',(315.70512949888,-71.2620589084766,478.668692955651));
#49907=CARTESIAN_POINT('Ctrl Pts',(315.730336994929,-71.2215467313676,478.740602142178));
#49908=CARTESIAN_POINT('Ctrl Pts',(315.754497079091,-71.1799959836181,478.809506878454));
#49909=CARTESIAN_POINT('Ctrl Pts',(315.777580511676,-71.1375810950581,478.875336513486));
#49910=CARTESIAN_POINT('Ctrl Pts',(315.790769900609,-71.1133461178848,478.912950185394));
#49911=CARTESIAN_POINT('Ctrl Pts',(315.803608130977,-71.0888290106729,478.949560855386));
#49912=CARTESIAN_POINT('Ctrl Pts',(315.816092334926,-71.0640622089115,478.985162467871));
#49913=CARTESIAN_POINT('Ctrl Pts',(315.82507579462,-71.0462403624972,479.010780893534));
#49914=CARTESIAN_POINT('Ctrl Pts',(315.833875964576,-71.0282892411033,479.035876897032));
#49915=CARTESIAN_POINT('Ctrl Pts',(315.842490838639,-71.0102232726035,479.060445490101));
#49916=CARTESIAN_POINT('Ctrl Pts',(315.864152558303,-70.9647971941416,479.122222130333));
#49917=CARTESIAN_POINT('Ctrl Pts',(315.88464476293,-70.9186326263578,479.18067703009));
#49918=CARTESIAN_POINT('Ctrl Pts',(315.903975797339,-70.8719111276457,479.235820367005));
#49919=CARTESIAN_POINT('Ctrl Pts',(315.918792309151,-70.8361008537166,479.278085663597));
#49920=CARTESIAN_POINT('Ctrl Pts',(315.932927065217,-70.7999629729406,479.318406696052));
#49921=CARTESIAN_POINT('Ctrl Pts',(315.946389844957,-70.7635713397338,479.356806033605));
#49922=CARTESIAN_POINT('Ctrl Pts',(315.949045471411,-70.7563928382873,479.364380568625));
#49923=CARTESIAN_POINT('Ctrl Pts',(315.951674965504,-70.7492044430815,479.37188037315));
#49924=CARTESIAN_POINT('Ctrl Pts',(315.954278375387,-70.7420068815996,479.379305546621));
#49925=CARTESIAN_POINT('Ctrl Pts',(317.115916695644,-72.0120079574161,481.0934972414));
#49926=CARTESIAN_POINT('Ctrl Pts',(317.115914706685,-71.975324917565,481.047447571311));
#49927=CARTESIAN_POINT('Ctrl Pts',(317.11386559519,-71.9392458075248,481.000577558259));
#49928=CARTESIAN_POINT('Ctrl Pts',(317.10972316475,-71.9036114492898,480.953288210959));
#49929=CARTESIAN_POINT('Ctrl Pts',(317.105609060625,-71.8682207620356,480.906322232516));
#49930=CARTESIAN_POINT('Ctrl Pts',(317.099430137655,-71.833268755692,480.858942794064));
#49931=CARTESIAN_POINT('Ctrl Pts',(317.091173129388,-71.7986331412772,480.811521171906));
#49932=CARTESIAN_POINT('Ctrl Pts',(317.082924470151,-71.7640325484783,480.764147499867));
#49933=CARTESIAN_POINT('Ctrl Pts',(317.072601907592,-71.7297478280276,480.716731922374));
#49934=CARTESIAN_POINT('Ctrl Pts',(317.060224668629,-71.6956899506149,480.669620323073));
#49935=CARTESIAN_POINT('Ctrl Pts',(317.053441419845,-71.6770247978915,480.643801180401));
#49936=CARTESIAN_POINT('Ctrl Pts',(317.046041620099,-71.6584283466728,480.618072895536));
#49937=CARTESIAN_POINT('Ctrl Pts',(317.038032573823,-71.6398898461305,480.592488983963));
#49938=CARTESIAN_POINT('Ctrl Pts',(317.016944480046,-71.5910773378187,480.525125666554));
#49939=CARTESIAN_POINT('Ctrl Pts',(316.991626974743,-71.5425836661291,480.458809113957));
#49940=CARTESIAN_POINT('Ctrl Pts',(316.96220235342,-71.4947553753167,480.393822217968));
#49941=CARTESIAN_POINT('Ctrl Pts',(316.933346129845,-71.4478509873964,480.330090679011));
#49942=CARTESIAN_POINT('Ctrl Pts',(316.900539885927,-71.4015866110813,480.267638101397));
#49943=CARTESIAN_POINT('Ctrl Pts',(316.863945856163,-71.3562721759521,480.206734254986));
#49944=CARTESIAN_POINT('Ctrl Pts',(316.845875461435,-71.3338955824212,480.176659498195));
#49945=CARTESIAN_POINT('Ctrl Pts',(316.826882164448,-71.3117503575587,480.146962423224));
#49946=CARTESIAN_POINT('Ctrl Pts',(316.806989910488,-71.289872130623,480.11767552603));
#49947=CARTESIAN_POINT('Ctrl Pts',(316.769937888749,-71.2491209647852,480.063124706718));
#49948=CARTESIAN_POINT('Ctrl Pts',(316.729764532366,-71.2092859907826,480.010003979968));
#49949=CARTESIAN_POINT('Ctrl Pts',(316.686645350494,-71.1706830835551,479.958438407935));
#49950=CARTESIAN_POINT('Ctrl Pts',(316.642896925465,-71.1315168396827,479.906120333606));
#49951=CARTESIAN_POINT('Ctrl Pts',(316.596115949078,-71.0936188702458,479.855403656897));
#49952=CARTESIAN_POINT('Ctrl Pts',(316.546521056654,-71.0572796433875,479.806429791048));
#49953=CARTESIAN_POINT('Ctrl Pts',(316.511418123213,-71.0315589814536,479.771766416068));
#49954=CARTESIAN_POINT('Ctrl Pts',(316.474906255075,-71.0066183661931,479.737976403483));
#49955=CARTESIAN_POINT('Ctrl Pts',(316.437073728139,-70.9825493079024,479.705110614392));
#49956=CARTESIAN_POINT('Ctrl Pts',(316.394280186412,-70.9553240513913,479.667935103509));
#49957=CARTESIAN_POINT('Ctrl Pts',(316.349795700217,-70.9292507855694,479.631914971486));
#49958=CARTESIAN_POINT('Ctrl Pts',(316.303781551238,-70.904190840024,479.597332522048));
#49959=CARTESIAN_POINT('Ctrl Pts',(316.256731387022,-70.8785666661709,479.561971443747));
#49960=CARTESIAN_POINT('Ctrl Pts',(316.208081773002,-70.8540025583256,479.528113523605));
#49961=CARTESIAN_POINT('Ctrl Pts',(316.158030950496,-70.8303782654384,479.496020534418));
#49962=CARTESIAN_POINT('Ctrl Pts',(316.106578421861,-70.8060923587252,479.463028760008));
#49963=CARTESIAN_POINT('Ctrl Pts',(316.053645043201,-70.7828005038837,479.431902289659));
#49964=CARTESIAN_POINT('Ctrl Pts',(315.999474742825,-70.7603900681349,479.402882556391));
#49965=CARTESIAN_POINT('Ctrl Pts',(315.984507093301,-70.7541979011052,479.394864192198));
#49966=CARTESIAN_POINT('Ctrl Pts',(315.969445175518,-70.7480730855507,479.387006414855));
#49967=CARTESIAN_POINT('Ctrl Pts',(315.954294505778,-70.7420133331691,479.379313736668));
#49968=CARTESIAN_POINT('Origin',(319.112977972408,-69.4720072687901,479.096520917133));
#49969=CARTESIAN_POINT('',(305.305026691757,-70.7420844489581,470.816561545459));
#49970=CARTESIAN_POINT('Origin',(306.683384790848,-69.47200726879,469.102280889483));
#49971=CARTESIAN_POINT('',(315.954278084408,-70.7420071496971,479.379305908523));
#49972=CARTESIAN_POINT('Origin',(306.683384790848,-69.47200726879,469.102280889483));
#49973=CARTESIAN_POINT('Origin',(306.683384790848,-69.47200726879,469.102280889483));
#49974=CARTESIAN_POINT('Origin',(306.683409153898,-69.4721780198136,469.102247046603));
#49975=CARTESIAN_POINT('Ctrl Pts',(304.480558603038,-69.4654490974856,473.087728863913));
#49976=CARTESIAN_POINT('Ctrl Pts',(304.498705664228,-69.4642164587728,473.056187095803));
#49977=CARTESIAN_POINT('Ctrl Pts',(304.613843052118,-69.4612105224026,472.854094590153));
#49978=CARTESIAN_POINT('Ctrl Pts',(304.816679229658,-69.513317227736,472.474231273923));
#49979=CARTESIAN_POINT('Ctrl Pts',(305.059765686868,-69.7138478877062,471.964996701443));
#49980=CARTESIAN_POINT('Ctrl Pts',(305.260591333288,-70.0353627268994,471.494352561143));
#49981=CARTESIAN_POINT('Ctrl Pts',(305.400342602498,-70.4245592719201,471.129965573733));
#49982=CARTESIAN_POINT('Ctrl Pts',(305.464816219258,-70.7132164602071,470.948704299693));
#49983=CARTESIAN_POINT('Ctrl Pts',(305.487849475208,-70.840784784687,470.882493350613));
#49984=CARTESIAN_POINT('Ctrl Pts',(303.098473769598,-69.6040686792588,472.138397726133));
#49985=CARTESIAN_POINT('Ctrl Pts',(303.114007019468,-69.6011683474859,472.110406731753));
#49986=CARTESIAN_POINT('Ctrl Pts',(303.212744305738,-69.5865972268538,471.930677833983));
#49987=CARTESIAN_POINT('Ctrl Pts',(303.389433235448,-69.6065541544155,471.587319568593));
#49988=CARTESIAN_POINT('Ctrl Pts',(303.613137828168,-69.7486471104222,471.105944697023));
#49989=CARTESIAN_POINT('Ctrl Pts',(303.813452001428,-70.0138432058711,470.636006546653));
#49990=CARTESIAN_POINT('Ctrl Pts',(303.966817657268,-70.3700332044193,470.250664139543));
#49991=CARTESIAN_POINT('Ctrl Pts',(304.043356984828,-70.653644403435,470.050648159123));
#49992=CARTESIAN_POINT('Ctrl Pts',(304.071326011608,-70.78193644975,469.976635184693));
#49993=CARTESIAN_POINT('Ctrl Pts',(302.085667889648,-68.419135632178,471.505330697043));
#49994=CARTESIAN_POINT('Ctrl Pts',(302.110606322998,-68.414325499387,471.465855536483));
#49995=CARTESIAN_POINT('Ctrl Pts',(302.269644108638,-68.389321427153,471.212527796443));
#49996=CARTESIAN_POINT('Ctrl Pts',(302.560567421638,-68.410944983966,470.729926704453));
#49997=CARTESIAN_POINT('Ctrl Pts',(302.943787016688,-68.6097419631934,470.052830454643));
#49998=CARTESIAN_POINT('Ctrl Pts',(303.300284786528,-68.9946417969067,469.388700136083));
#49999=CARTESIAN_POINT('Ctrl Pts',(303.582351736368,-69.5228226663637,468.840440988033));
#50000=CARTESIAN_POINT('Ctrl Pts',(303.726036985068,-69.9489645106605,468.554258016843));
#50001=CARTESIAN_POINT('Ctrl Pts',(303.778845690928,-70.1425212887321,468.448172524813));
#50002=CARTESIAN_POINT('Ctrl Pts',(302.153517964228,-66.742926046005,471.633182901113));
#50003=CARTESIAN_POINT('Ctrl Pts',(302.193274540738,-66.737305414815,471.575254910373));
#50004=CARTESIAN_POINT('Ctrl Pts',(302.446959418678,-66.710328544982,471.204060407683));
#50005=CARTESIAN_POINT('Ctrl Pts',(302.912262528458,-66.766264527055,470.504270319133));
#50006=CARTESIAN_POINT('Ctrl Pts',(303.521853466188,-67.097079350092,469.545342858733));
#50007=CARTESIAN_POINT('Ctrl Pts',(304.081529296598,-67.693627607904,468.628519370473));
#50008=CARTESIAN_POINT('Ctrl Pts',(304.516986927068,-68.4779934089828,467.889812007953));
#50009=CARTESIAN_POINT('Ctrl Pts',(304.735736195578,-69.0941315197382,467.510571937363));
#50010=CARTESIAN_POINT('Ctrl Pts',(304.815841535928,-69.3716532420849,467.370670606613));
#50011=CARTESIAN_POINT('Ctrl Pts',(304.36560734514,-69.4720072829635,472.883816394761));
#50012=CARTESIAN_POINT('Ctrl Pts',(304.437924386038,-69.4720061785358,472.755478620527));
#50013=CARTESIAN_POINT('Ctrl Pts',(304.578280640235,-69.4970261445459,472.495428198348));
#50014=CARTESIAN_POINT('Ctrl Pts',(304.771191553278,-69.6083606205034,472.107646255653));
#50015=CARTESIAN_POINT('Ctrl Pts',(304.942919591518,-69.7913397669247,471.732484512733));
#50016=CARTESIAN_POINT('Ctrl Pts',(305.091118069088,-70.0432002703421,471.381409217703));
#50017=CARTESIAN_POINT('Ctrl Pts',(305.213936884918,-70.3602758159736,471.067167469123));
#50018=CARTESIAN_POINT('Ctrl Pts',(305.277815958598,-70.609423919947,470.892937814703));
#50019=CARTESIAN_POINT('Ctrl Pts',(305.305042216108,-70.742010890829,470.816601123963));
#50020=CARTESIAN_POINT('Origin',(317.464909153118,-72.0120072687901,483.416551570203));
#50021=CARTESIAN_POINT('Origin',(314.575917770968,-72.0120072687901,481.093605606543));
#50022=CARTESIAN_POINT('Origin',(314.575917770968,-72.0120072687901,481.093605606543));
#50023=CARTESIAN_POINT('Origin',(314.575917770968,-72.0120072687901,481.093605606543));
#50024=CARTESIAN_POINT('Origin',(314.575917770968,-72.01200726879,402.251606455353));
#50025=CARTESIAN_POINT('Origin',(263.115917770968,-69.47200726879,445.000000551893));
#50026=CARTESIAN_POINT('Origin',(306.683384790848,-69.47200726879,420.897720214303));
#50027=CARTESIAN_POINT('Origin',(306.683384790848,-69.47200726879,420.897720214303));
#50028=CARTESIAN_POINT('Origin',(306.683384790848,-69.47200726879,420.897720214303));
#50029=CARTESIAN_POINT('Origin',(208.951764595088,-69.47200726879,499.480603520313));
#50030=CARTESIAN_POINT('Origin',(263.115917770968,-69.47200726879,445.000000551893));
#50031=CARTESIAN_POINT('Origin',(239.013637433378,-69.4720072687899,401.432533532013));
#50032=CARTESIAN_POINT('Ctrl Pts',(235.028190410038,-69.46544846321,486.364643478553));
#50033=CARTESIAN_POINT('Ctrl Pts',(235.058784398358,-69.4642529784631,486.382245155523));
#50034=CARTESIAN_POINT('Ctrl Pts',(235.258976493428,-69.461131317104,486.496332464443));
#50035=CARTESIAN_POINT('Ctrl Pts',(235.636888941828,-69.5121743079281,486.698315147843));
#50036=CARTESIAN_POINT('Ctrl Pts',(236.146870785568,-69.711509521041,486.942061181483));
#50037=CARTESIAN_POINT('Ctrl Pts',(236.619881789448,-70.0335847626079,487.144032803713));
#50038=CARTESIAN_POINT('Ctrl Pts',(236.985786004388,-70.4242464530176,487.284367991343));
#50039=CARTESIAN_POINT('Ctrl Pts',(237.167315497998,-70.713413234505,487.348935251613));
#50040=CARTESIAN_POINT('Ctrl Pts',(237.233421929898,-70.840779768824,487.371932164383));
#50041=CARTESIAN_POINT('Ctrl Pts',(235.977522050648,-69.6040686220959,484.982557637913));
#50042=CARTESIAN_POINT('Ctrl Pts',(236.004671893388,-69.6012555491032,484.997624146153));
#50043=CARTESIAN_POINT('Ctrl Pts',(236.182698522748,-69.5867035136386,485.095456441663));
#50044=CARTESIAN_POINT('Ctrl Pts',(236.524196098828,-69.605895880883,485.271347646443));
#50045=CARTESIAN_POINT('Ctrl Pts',(237.006005570248,-69.7468138148857,485.495488520553));
#50046=CARTESIAN_POINT('Ctrl Pts',(237.478127991128,-70.0122251216762,485.696827627373));
#50047=CARTESIAN_POINT('Ctrl Pts',(237.865067852528,-70.3697189200575,485.850830120423));
#50048=CARTESIAN_POINT('Ctrl Pts',(238.065383438968,-70.653842506004,485.927482824733));
#50049=CARTESIAN_POINT('Ctrl Pts',(238.139279526348,-70.781931585494,485.955407815003));
#50050=CARTESIAN_POINT('Ctrl Pts',(236.610590348658,-68.419135189814,483.969751425023));
#50051=CARTESIAN_POINT('Ctrl Pts',(236.648879211058,-68.41446975451,483.993940563573));
#50052=CARTESIAN_POINT('Ctrl Pts',(236.899811351788,-68.389529900869,484.151505778333));
#50053=CARTESIAN_POINT('Ctrl Pts',(237.379808367058,-68.410079767087,484.441021758033));
#50054=CARTESIAN_POINT('Ctrl Pts',(238.057492885838,-68.6071111008896,484.824821137953));
#50055=CARTESIAN_POINT('Ctrl Pts',(238.724680693938,-68.9922445608702,485.183064252343));
#50056=CARTESIAN_POINT('Ctrl Pts',(239.275210865108,-69.5223481989856,485.466301413533));
#50057=CARTESIAN_POINT('Ctrl Pts',(239.561823319288,-69.9492631288263,485.610200564473));
#50058=CARTESIAN_POINT('Ctrl Pts',(239.667741277698,-70.1425137073577,485.662926108393));
#50059=CARTESIAN_POINT('Ctrl Pts',(236.482739132008,-66.742924819268,484.037602324843));
#50060=CARTESIAN_POINT('Ctrl Pts',(236.538926325478,-66.737473314687,484.076164315743));
#50061=CARTESIAN_POINT('Ctrl Pts',(236.906627390308,-66.710484421782,484.327495017863));
#50062=CARTESIAN_POINT('Ctrl Pts',(237.602758556818,-66.764646425836,484.790543958523));
#50063=CARTESIAN_POINT('Ctrl Pts',(238.562786312978,-67.092908761381,485.401124149403));
#50064=CARTESIAN_POINT('Ctrl Pts',(239.483982940058,-67.690059702463,485.963601145843));
#50065=CARTESIAN_POINT('Ctrl Pts',(240.225755093378,-68.4773127599914,486.400868152653));
#50066=CARTESIAN_POINT('Ctrl Pts',(240.605561769818,-69.094559414416,486.619942017203));
#50067=CARTESIAN_POINT('Ctrl Pts',(240.745242209038,-69.3716421412076,486.699921112973));
#50068=CARTESIAN_POINT('',(237.299356354755,-70.7420814892879,487.189107554724));
#50069=CARTESIAN_POINT('Ctrl Pts',(235.232102033643,-69.4720072796082,486.249690185527));
#50070=CARTESIAN_POINT('Ctrl Pts',(235.3592580076,-69.4720058497161,486.321341955001));
#50071=CARTESIAN_POINT('Ctrl Pts',(235.488356422264,-69.4843168520743,486.391048411963));
#50072=CARTESIAN_POINT('Ctrl Pts',(235.658418468521,-69.5166114182826,486.479309551096));
#50073=CARTESIAN_POINT('Ctrl Pts',(235.699575114172,-69.5256727717999,486.500398420692));
#50074=CARTESIAN_POINT('Ctrl Pts',(235.828178647505,-69.5579244915859,486.565443702623));
#50075=CARTESIAN_POINT('Ctrl Pts',(235.915403941424,-69.5855055087001,486.608325495863));
#50076=CARTESIAN_POINT('Ctrl Pts',(236.082685935217,-69.6496600928298,486.688345395098));
#50077=CARTESIAN_POINT('Ctrl Pts',(236.162832376958,-69.6855216028279,486.725675808643));
#50078=CARTESIAN_POINT('Ctrl Pts',(236.28711143786,-69.7495837444741,486.782105481196));
#50079=CARTESIAN_POINT('Ctrl Pts',(236.33206025476,-69.7745536342549,486.802204687413));
#50080=CARTESIAN_POINT('Ctrl Pts',(236.492448571889,-69.8703147051983,486.872903627949));
#50081=CARTESIAN_POINT('Ctrl Pts',(236.604898071057,-69.9501642898247,486.92049203298));
#50082=CARTESIAN_POINT('Ctrl Pts',(236.717004498143,-70.0443954690103,486.966335815599));
#50083=CARTESIAN_POINT('Ctrl Pts',(236.722327705171,-70.0489065580006,486.968508642302));
#50084=CARTESIAN_POINT('Ctrl Pts',(236.839139822294,-70.1487082562837,487.016102550549));
#50085=CARTESIAN_POINT('Ctrl Pts',(236.944250966748,-70.2548440769946,487.057176136868));
#50086=CARTESIAN_POINT('Ctrl Pts',(237.066131244566,-70.4011757050274,487.103468011324));
#50087=CARTESIAN_POINT('Ctrl Pts',(237.091327483615,-70.4328767762969,487.11295359292));
#50088=CARTESIAN_POINT('Ctrl Pts',(237.182331506607,-70.5529932331032,487.146934631606));
#50089=CARTESIAN_POINT('Ctrl Pts',(237.243714297159,-70.6454659295432,487.169284956413));
#50090=CARTESIAN_POINT('Ctrl Pts',(237.299306537109,-70.7420200540544,487.189112906131));
#50091=CARTESIAN_POINT('Origin',(239.013668569868,-69.4721721185271,488.567490430283));
#50092=CARTESIAN_POINT('Origin',(235.232099195168,-66.932007290493,486.249688566713));
#50093=CARTESIAN_POINT('Origin',(224.680024455158,-72.01200726879,499.373047478893));
#50094=CARTESIAN_POINT('',(228.736601009321,-70.7420092778759,497.838377092546));
#50095=CARTESIAN_POINT('Origin',(227.022312716318,-72.01200726879,496.460000551893));
#50096=CARTESIAN_POINT('',(228.736612414338,-70.742007149697,497.838360865333));
#50097=CARTESIAN_POINT('Origin',(229.003814201928,-69.47200726879,501.016441204783));
#50098=CARTESIAN_POINT('Origin',(239.013637433378,-69.47200726879,488.567467571773));
#50099=CARTESIAN_POINT('Ctrl Pts',(232.667503020318,-72.01200726879,496.460000551893));
#50100=CARTESIAN_POINT('Ctrl Pts',(232.552467855573,-72.0120072687895,496.50034510223));
#50101=CARTESIAN_POINT('Ctrl Pts',(232.439630484044,-72.0095636111055,496.539900696401));
#50102=CARTESIAN_POINT('Ctrl Pts',(232.32901983994,-72.0049345804185,496.578681378017));
#50103=CARTESIAN_POINT('Ctrl Pts',(232.214621370972,-72.0001470301093,496.618790091227));
#50104=CARTESIAN_POINT('Ctrl Pts',(232.102604351893,-71.9930221141204,496.658069591567));
#50105=CARTESIAN_POINT('Ctrl Pts',(231.992972675035,-71.9838027053761,496.6965128071));
#50106=CARTESIAN_POINT('Ctrl Pts',(231.94065912929,-71.9794034297751,496.714856966124));
#50107=CARTESIAN_POINT('Ctrl Pts',(231.888888351699,-71.9745266060022,496.733010412023));
#50108=CARTESIAN_POINT('Ctrl Pts',(231.83765902232,-71.9691951485491,496.750970975055));
#50109=CARTESIAN_POINT('Ctrl Pts',(231.719354046327,-71.9568831008675,496.792447683885));
#50110=CARTESIAN_POINT('Ctrl Pts',(231.603941821324,-71.9421444368137,496.83289995809));
#50111=CARTESIAN_POINT('Ctrl Pts',(231.491767776884,-71.9253093502902,496.872233052362));
#50112=CARTESIAN_POINT('Ctrl Pts',(231.377934231753,-71.9082252058153,496.912148039687));
#50113=CARTESIAN_POINT('Ctrl Pts',(231.267435458371,-71.8889826584263,496.950910545216));
#50114=CARTESIAN_POINT('Ctrl Pts',(231.160592692157,-71.8679429935163,496.988389592098));
#50115=CARTESIAN_POINT('Ctrl Pts',(231.139204181572,-71.8637311304995,496.995892402249));
#50116=CARTESIAN_POINT('Ctrl Pts',(231.117962057352,-71.8594472855261,497.003343675825));
#50117=CARTESIAN_POINT('Ctrl Pts',(231.096868706623,-71.8550944057315,497.010742209328));
#50118=CARTESIAN_POINT('Ctrl Pts',(230.994786588947,-71.834028469214,497.046547709236));
#50119=CARTESIAN_POINT('Ctrl Pts',(230.896191382266,-71.8113504463176,497.081119958007));
#50120=CARTESIAN_POINT('Ctrl Pts',(230.800915719752,-71.7872977520841,497.114529086895));
#50121=CARTESIAN_POINT('Ctrl Pts',(230.702607866525,-71.7624795700636,497.149001476302));
#50122=CARTESIAN_POINT('Ctrl Pts',(230.607833795941,-71.7361978239251,497.182235199856));
#50123=CARTESIAN_POINT('Ctrl Pts',(230.516397501224,-71.7086604136538,497.214297533498));
#50124=CARTESIAN_POINT('Ctrl Pts',(230.496534912513,-71.7026784974344,497.221262393002));
#50125=CARTESIAN_POINT('Ctrl Pts',(230.476829796947,-71.6966371365143,497.228171951769));
#50126=CARTESIAN_POINT('Ctrl Pts',(230.457280101594,-71.6905381477013,497.235026864256));
#50127=CARTESIAN_POINT('Ctrl Pts',(230.366315753107,-71.6621596725492,497.266922637414));
#50128=CARTESIAN_POINT('Ctrl Pts',(230.278721835742,-71.6325417447297,497.297639767496));
#50129=CARTESIAN_POINT('Ctrl Pts',(230.194254442441,-71.6018271779252,497.327260296549));
#50130=CARTESIAN_POINT('Ctrl Pts',(230.107506337049,-71.5702832841915,497.357680612315));
#50131=CARTESIAN_POINT('Ctrl Pts',(230.024055457235,-71.5375825442999,497.386943973369));
#50132=CARTESIAN_POINT('Ctrl Pts',(229.943641520358,-71.5038254269623,497.415142400406));
#50133=CARTESIAN_POINT('Ctrl Pts',(229.932984397381,-71.4993516533258,497.418879490223));
#50134=CARTESIAN_POINT('Ctrl Pts',(229.922380625256,-71.4948592522483,497.422597884436));
#50135=CARTESIAN_POINT('Ctrl Pts',(229.911829609023,-71.4903483914863,497.426297806007));
#50136=CARTESIAN_POINT('Ctrl Pts',(229.824112674067,-71.4528468967154,497.457057476225));
#50137=CARTESIAN_POINT('Ctrl Pts',(229.740045190858,-71.4140777953039,497.486542947253));
#50138=CARTESIAN_POINT('Ctrl Pts',(229.659402575902,-71.3741434343248,497.514821730231));
#50139=CARTESIAN_POINT('Ctrl Pts',(229.585884356645,-71.337737086292,497.540602215752));
#50140=CARTESIAN_POINT('Ctrl Pts',(229.515212470564,-71.3003613442696,497.565379706035));
#50141=CARTESIAN_POINT('Ctrl Pts',(229.447226075572,-71.2620580055471,497.5892128494));
#50142=CARTESIAN_POINT('Ctrl Pts',(229.354619849438,-71.209883925015,497.621676660199));
#50143=CARTESIAN_POINT('Ctrl Pts',(229.267002875685,-71.1559856710929,497.652393646307));
#50144=CARTESIAN_POINT('Ctrl Pts',(229.184502681344,-71.1007413457377,497.681324771646));
#50145=CARTESIAN_POINT('Ctrl Pts',(229.139999322598,-71.0709407125436,497.696931186396));
#50146=CARTESIAN_POINT('Ctrl Pts',(229.096984178731,-71.0407484336903,497.712017366799));
#50147=CARTESIAN_POINT('Ctrl Pts',(229.055472371791,-71.0102237227464,497.726573248913));
#50148=CARTESIAN_POINT('Ctrl Pts',(228.974165797026,-70.9504368843627,497.755082943012));
#50149=CARTESIAN_POINT('Ctrl Pts',(228.898627668183,-70.8893746621778,497.781559283438));
#50150=CARTESIAN_POINT('Ctrl Pts',(228.82879483944,-70.8274387196506,497.806041823638));
#50151=CARTESIAN_POINT('Ctrl Pts',(228.796879010488,-70.7991320194465,497.817231124993));
#50152=CARTESIAN_POINT('Ctrl Pts',(228.766154363183,-70.7706425598328,497.828003538254));
#50153=CARTESIAN_POINT('Ctrl Pts',(228.736612293562,-70.7420072391727,497.838360768221));
#50154=CARTESIAN_POINT('Origin',(239.013637433378,-69.47200726879,488.567467571773));
#50155=CARTESIAN_POINT('Ctrl Pts',(232.828215541778,-74.713507444107,498.994794772563));
#50156=CARTESIAN_POINT('Ctrl Pts',(232.708581879358,-74.744487732072,498.992935002363));
#50157=CARTESIAN_POINT('Ctrl Pts',(232.135343545468,-74.879297233076,498.981813429663));
#50158=CARTESIAN_POINT('Ctrl Pts',(231.115092555868,-75.007840422924,498.944324337233));
#50159=CARTESIAN_POINT('Ctrl Pts',(229.794873524148,-74.948821572214,498.864713031993));
#50160=CARTESIAN_POINT('Ctrl Pts',(228.602549223458,-74.694184459517,498.770637037043));
#50161=CARTESIAN_POINT('Ctrl Pts',(227.544153995848,-74.277385902565,498.671516955493));
#50162=CARTESIAN_POINT('Ctrl Pts',(226.618188533358,-73.717781829921,498.573974289063));
#50163=CARTESIAN_POINT('Ctrl Pts',(226.002925806248,-73.179135190463,498.503623109783));
#50164=CARTESIAN_POINT('Ctrl Pts',(225.700915179718,-72.841170440473,498.467827978703));
#50165=CARTESIAN_POINT('Ctrl Pts',(225.638265364858,-72.767200936835,498.460354730143));
#50166=CARTESIAN_POINT('Ctrl Pts',(232.796568792498,-73.034824311939,499.102763601033));
#50167=CARTESIAN_POINT('Ctrl Pts',(232.700627839608,-73.066583901593,499.119930810033));
#50168=CARTESIAN_POINT('Ctrl Pts',(232.239472322888,-73.209004644328,499.198942363853));
#50169=CARTESIAN_POINT('Ctrl Pts',(231.407183411038,-73.381806588117,499.313593076103));
#50170=CARTESIAN_POINT('Ctrl Pts',(230.309431538318,-73.435351583061,499.415978913903));
#50171=CARTESIAN_POINT('Ctrl Pts',(229.301912439328,-73.326904152345,499.474828842763));
#50172=CARTESIAN_POINT('Ctrl Pts',(228.394849201738,-73.078553798327,499.502527799073));
#50173=CARTESIAN_POINT('Ctrl Pts',(227.591135930828,-72.703469484999,499.508897708423));
#50174=CARTESIAN_POINT('Ctrl Pts',(227.050979790138,-72.31828963445,499.503395046963));
#50175=CARTESIAN_POINT('Ctrl Pts',(226.784203935658,-72.069395060257,499.498324453983));
#50176=CARTESIAN_POINT('Ctrl Pts',(226.728793427818,-72.014632724146,499.497177704013));
#50177=CARTESIAN_POINT('Ctrl Pts',(232.774487437958,-71.863532363329,497.895184339653));
#50178=CARTESIAN_POINT('Ctrl Pts',(232.694803909168,-71.881299175708,497.925633863583));
#50179=CARTESIAN_POINT('Ctrl Pts',(232.313470385268,-71.960042879053,498.068730506413));
#50180=CARTESIAN_POINT('Ctrl Pts',(231.638597324018,-72.047682887232,498.300987160673));
#50181=CARTESIAN_POINT('Ctrl Pts',(230.772193181568,-72.052539058419,498.561581886413));
#50182=CARTESIAN_POINT('Ctrl Pts',(229.995069126148,-71.958291489615,498.767069706243));
#50183=CARTESIAN_POINT('Ctrl Pts',(229.309457180988,-71.779984113588,498.927010515113));
#50184=CARTESIAN_POINT('Ctrl Pts',(228.712998830268,-71.526452518351,499.049965226743));
#50185=CARTESIAN_POINT('Ctrl Pts',(228.318711996458,-71.274222914498,499.121996638453));
#50186=CARTESIAN_POINT('Ctrl Pts',(228.125712481478,-71.113515579462,499.154902555743));
#50187=CARTESIAN_POINT('Ctrl Pts',(228.085699392628,-71.078244434764,499.161627305873));
#50188=CARTESIAN_POINT('Ctrl Pts',(232.777480917018,-72.022320298527,496.220233067973));
#50189=CARTESIAN_POINT('Ctrl Pts',(232.695200683688,-72.021150461685,496.248891048053));
#50190=CARTESIAN_POINT('Ctrl Pts',(232.305363184468,-72.009654141941,496.385012840253));
#50191=CARTESIAN_POINT('Ctrl Pts',(231.646794450228,-71.942527322552,496.617737847513));
#50192=CARTESIAN_POINT('Ctrl Pts',(230.858125249948,-71.771639917819,496.901630898333));
#50193=CARTESIAN_POINT('Ctrl Pts',(230.195161865978,-71.549628732325,497.144473472413));
#50194=CARTESIAN_POINT('Ctrl Pts',(229.645578188088,-71.293762522114,497.349195293073));
#50195=CARTESIAN_POINT('Ctrl Pts',(229.195806366078,-71.013440752079,497.519520532373));
#50196=CARTESIAN_POINT('Ctrl Pts',(228.915696291618,-70.780263637391,497.627313411293));
#50197=CARTESIAN_POINT('Ctrl Pts',(228.783195868548,-70.644919903199,497.678773977973));
#50198=CARTESIAN_POINT('Ctrl Pts',(228.755923515418,-70.615733806332,497.689386467923));
#50199=CARTESIAN_POINT('',(227.022399636625,-72.0120079573874,499.000000348522));
#50200=CARTESIAN_POINT('Ctrl Pts',(227.022421081461,-72.012007957416,498.999999476569));
#50201=CARTESIAN_POINT('Ctrl Pts',(227.06847075155,-71.9753249175649,498.99999748761));
#50202=CARTESIAN_POINT('Ctrl Pts',(227.115340764603,-71.9392458075247,498.997948376115));
#50203=CARTESIAN_POINT('Ctrl Pts',(227.162630111902,-71.9036114492896,498.993805945675));
#50204=CARTESIAN_POINT('Ctrl Pts',(227.209596090345,-71.8682207620356,498.98969184155));
#50205=CARTESIAN_POINT('Ctrl Pts',(227.256975528797,-71.8332687556922,498.98351291858));
#50206=CARTESIAN_POINT('Ctrl Pts',(227.304397150955,-71.7986331412776,498.975255910314));
#50207=CARTESIAN_POINT('Ctrl Pts',(227.351770822992,-71.7640325484796,498.967007251077));
#50208=CARTESIAN_POINT('Ctrl Pts',(227.399186400484,-71.7297478280298,498.956684688518));
#50209=CARTESIAN_POINT('Ctrl Pts',(227.446297999784,-71.6956899506178,498.944307449555));
#50210=CARTESIAN_POINT('Ctrl Pts',(227.472117142457,-71.6770247978935,498.937524200771));
#50211=CARTESIAN_POINT('Ctrl Pts',(227.497845427324,-71.6584283466738,498.930124401024));
#50212=CARTESIAN_POINT('Ctrl Pts',(227.523429338898,-71.6398898461305,498.922115354748));
#50213=CARTESIAN_POINT('Ctrl Pts',(227.590792656308,-71.591077337818,498.90102726097));
#50214=CARTESIAN_POINT('Ctrl Pts',(227.657109208906,-71.5425836661277,498.875709755667));
#50215=CARTESIAN_POINT('Ctrl Pts',(227.722096104895,-71.4947553753147,498.846285134344));
#50216=CARTESIAN_POINT('Ctrl Pts',(227.785827643853,-71.4478509873942,498.817428910768));
#50217=CARTESIAN_POINT('Ctrl Pts',(227.848280221467,-71.4015866110791,498.78462266685));
#50218=CARTESIAN_POINT('Ctrl Pts',(227.909184067879,-71.3562721759498,498.748028637086));
#50219=CARTESIAN_POINT('Ctrl Pts',(227.939258824668,-71.3338955824197,498.729958242358));
#50220=CARTESIAN_POINT('Ctrl Pts',(227.968955899638,-71.311750357558,498.710964945372));
#50221=CARTESIAN_POINT('Ctrl Pts',(227.998242796831,-71.2898721306231,498.691072691413));
#50222=CARTESIAN_POINT('Ctrl Pts',(228.052793616142,-71.2491209647857,498.654020669675));
#50223=CARTESIAN_POINT('Ctrl Pts',(228.105914342892,-71.2092859907835,498.613847313292));
#50224=CARTESIAN_POINT('Ctrl Pts',(228.157479914924,-71.1706830835565,498.570728131421));
#50225=CARTESIAN_POINT('Ctrl Pts',(228.209797989254,-71.1315168396836,498.526979706391));
#50226=CARTESIAN_POINT('Ctrl Pts',(228.260514665963,-71.0936188702463,498.480198730004));
#50227=CARTESIAN_POINT('Ctrl Pts',(228.309488531813,-71.0572796433875,498.430603837579));
#50228=CARTESIAN_POINT('Ctrl Pts',(228.344151906793,-71.0315589814536,498.395500904138));
#50229=CARTESIAN_POINT('Ctrl Pts',(228.377941919378,-71.0066183661931,498.358989036));
#50230=CARTESIAN_POINT('Ctrl Pts',(228.410807708469,-70.9825493079025,498.321156509064));
#50231=CARTESIAN_POINT('Ctrl Pts',(228.447983219353,-70.9553240513908,498.278362967336));
#50232=CARTESIAN_POINT('Ctrl Pts',(228.484003351377,-70.9292507855684,498.233878481141));
#50233=CARTESIAN_POINT('Ctrl Pts',(228.518585800815,-70.9041908400226,498.18786433216));
#50234=CARTESIAN_POINT('Ctrl Pts',(228.553946879116,-70.8785666661695,498.140814167944));
#50235=CARTESIAN_POINT('Ctrl Pts',(228.587804799258,-70.8540025583241,498.092164553924));
#50236=CARTESIAN_POINT('Ctrl Pts',(228.619897788445,-70.8303782654369,498.042113731418));
#50237=CARTESIAN_POINT('Ctrl Pts',(228.652889562856,-70.8060923587233,497.990661202781));
#50238=CARTESIAN_POINT('Ctrl Pts',(228.684016033206,-70.7828005038813,497.93772782412));
#50239=CARTESIAN_POINT('Ctrl Pts',(228.713035766474,-70.7603900681321,497.883557523744));
#50240=CARTESIAN_POINT('Ctrl Pts',(228.721054130665,-70.7541979011036,497.868589874222));
#50241=CARTESIAN_POINT('Ctrl Pts',(228.728911908006,-70.7480730855502,497.853527956442));
#50242=CARTESIAN_POINT('Ctrl Pts',(228.736604586192,-70.7420133331698,497.838377286705));
#50243=CARTESIAN_POINT('',(232.667503019844,-74.5520072687783,499.00000447072));
#50244=CARTESIAN_POINT('Ctrl Pts',(232.667503019828,-74.552007268779,499.000004766233));
#50245=CARTESIAN_POINT('Ctrl Pts',(232.248833705458,-74.551992484692,498.999983408163));
#50246=CARTESIAN_POINT('Ctrl Pts',(231.455510492608,-74.490207324118,499.000008510273));
#50247=CARTESIAN_POINT('Ctrl Pts',(230.386046693498,-74.254566710358,498.999998413173));
#50248=CARTESIAN_POINT('Ctrl Pts',(229.470698714398,-73.920471430072,499.000001148393));
#50249=CARTESIAN_POINT('Ctrl Pts',(228.690942526618,-73.517848718933,499.000000304633));
#50250=CARTESIAN_POINT('Ctrl Pts',(228.025995010608,-73.060368306828,499.000000944453));
#50251=CARTESIAN_POINT('Ctrl Pts',(227.462209463058,-72.553339670543,498.999999228903));
#50252=CARTESIAN_POINT('Ctrl Pts',(227.158361801518,-72.195521218722,499.000003377153));
#50253=CARTESIAN_POINT('Ctrl Pts',(227.022421081468,-72.012007957393,499.000000073513));
#50254=CARTESIAN_POINT('Origin',(232.667503019858,-74.552013924409,496.460000551893));
#50255=CARTESIAN_POINT('Origin',(305.864311867508,-74.5520072687901,496.460000551893));
#50256=CARTESIAN_POINT('',(293.56433252188,-74.5520072687791,499.000004766103));
#50257=CARTESIAN_POINT('',(293.564332522018,-74.5520072687791,499.000004766103));
#50258=CARTESIAN_POINT('Origin',(293.564332521738,-74.5520072687901,496.460000551893));
#50259=CARTESIAN_POINT('Origin',(220.615917770968,-69.47200726879,499.000000551893));
#50260=CARTESIAN_POINT('Ctrl Pts',(299.209414458968,-72.0120079557911,499.000000073343));
#50261=CARTESIAN_POINT('Ctrl Pts',(299.073473744338,-72.1955212182401,499.000003378503));
#50262=CARTESIAN_POINT('Ctrl Pts',(298.769626079658,-72.5533396718461,498.999999228283));
#50263=CARTESIAN_POINT('Ctrl Pts',(298.205840530728,-73.0603683052571,499.000000944623));
#50264=CARTESIAN_POINT('Ctrl Pts',(297.540893016148,-73.5178487195051,499.000000304583));
#50265=CARTESIAN_POINT('Ctrl Pts',(296.761136827618,-73.9204714296421,499.000001148393));
#50266=CARTESIAN_POINT('Ctrl Pts',(295.845788848668,-74.2545667103361,498.999998413213));
#50267=CARTESIAN_POINT('Ctrl Pts',(294.776325049528,-74.4902073240851,499.000008510113));
#50268=CARTESIAN_POINT('Ctrl Pts',(293.983001836448,-74.5519924854471,498.999983408503));
#50269=CARTESIAN_POINT('Ctrl Pts',(293.564332522018,-74.5520072687791,499.000004766103));
#50270=CARTESIAN_POINT('',(220.615917755701,-72.0120072687902,499.000000551894));
#50271=CARTESIAN_POINT('',(227.022421081468,-72.012007957393,499.000000073513));
#50272=CARTESIAN_POINT('',(220.615917770968,-85.47200726879,499.000000551893));
#50273=CARTESIAN_POINT('Origin',(220.615917770968,-69.47200726879,487.500000551893));
#50274=CARTESIAN_POINT('',(209.115917770968,-72.01200726879,487.500000551203));
#50275=CARTESIAN_POINT('Origin',(220.615917770968,-72.01200726879,487.500000551893));
#50276=CARTESIAN_POINT('',(209.115917770968,-85.47200726879,487.500000551893));
#50277=CARTESIAN_POINT('Origin',(220.615917770968,-72.01200726879,487.500000551893));
#50278=CARTESIAN_POINT('Origin',(220.615917745948,-72.01200726879,496.460000551893));
#50279=CARTESIAN_POINT('Origin',(211.655917770968,-72.01200726879,487.500000551893));
#50280=CARTESIAN_POINT('Origin',(211.655917770968,-72.01200726879,487.748394648433));
#50281=CARTESIAN_POINT('',(209.115918153386,-72.0120048639453,481.093519010876));
#50282=CARTESIAN_POINT('Origin',(211.655917770968,-72.01200726879,481.093605606543));
#50283=CARTESIAN_POINT('',(209.115917770968,-72.01200726879,487.500000551203));
#50284=CARTESIAN_POINT('Origin',(209.115917770968,-69.4720072687899,402.500000551893));
#50285=CARTESIAN_POINT('',(209.115913556758,-74.552007268779,475.448415302943));
#50286=CARTESIAN_POINT('Ctrl Pts',(209.115918249518,-72.012007955791,481.093497239893));
#50287=CARTESIAN_POINT('Ctrl Pts',(209.115914944358,-72.19552121824,480.957556525263));
#50288=CARTESIAN_POINT('Ctrl Pts',(209.115919094578,-72.553339671846,480.653708860583));
#50289=CARTESIAN_POINT('Ctrl Pts',(209.115917378238,-73.060368305257,480.089923311653));
#50290=CARTESIAN_POINT('Ctrl Pts',(209.115918018278,-73.517848719505,479.424975797073));
#50291=CARTESIAN_POINT('Ctrl Pts',(209.115917174468,-73.920471429642,478.645219608543));
#50292=CARTESIAN_POINT('Ctrl Pts',(209.115919909648,-74.254566710336,477.729871629593));
#50293=CARTESIAN_POINT('Ctrl Pts',(209.115909812748,-74.490207324085,476.660407830453));
#50294=CARTESIAN_POINT('Ctrl Pts',(209.115934914358,-74.551992485447,475.867084617373));
#50295=CARTESIAN_POINT('Ctrl Pts',(209.115913556758,-74.552007268779,475.448415302943));
#50296=CARTESIAN_POINT('',(209.115913852141,-74.5520072687782,414.551585800769));
#50297=CARTESIAN_POINT('',(209.115913556758,-74.552007268779,475.448415302943));
#50298=CARTESIAN_POINT('',(209.115918153252,-72.0120048645283,408.90648209161));
#50299=CARTESIAN_POINT('Ctrl Pts',(209.115913556628,-74.5520072687789,414.551585800753));
#50300=CARTESIAN_POINT('Ctrl Pts',(209.115934914698,-74.5519924846919,414.132916486383));
#50301=CARTESIAN_POINT('Ctrl Pts',(209.115909812588,-74.4902073241179,413.339593273533));
#50302=CARTESIAN_POINT('Ctrl Pts',(209.115919909688,-74.2545667103599,412.270129474423));
#50303=CARTESIAN_POINT('Ctrl Pts',(209.115917174468,-73.9204714300629,411.354781495313));
#50304=CARTESIAN_POINT('Ctrl Pts',(209.115918018228,-73.5178487189669,410.575025307573));
#50305=CARTESIAN_POINT('Ctrl Pts',(209.115917378408,-73.0603683067019,409.910077791393));
#50306=CARTESIAN_POINT('Ctrl Pts',(209.115919093958,-72.5533396710129,409.346292244473));
#50307=CARTESIAN_POINT('Ctrl Pts',(209.115914945708,-72.1955212177089,409.042444581383));
#50308=CARTESIAN_POINT('Ctrl Pts',(209.115918249348,-72.0120079562219,408.906503861543));
#50309=CARTESIAN_POINT('',(209.115918249348,-72.0120079562219,408.906503861543));
#50310=CARTESIAN_POINT('Origin',(211.655917770968,-72.01200726879,487.748394648433));
#50311=CARTESIAN_POINT('Origin',(211.655917770968,-72.0120072687899,408.906395497243));
#50312=CARTESIAN_POINT('Origin',(211.655917770968,-72.0120072687899,408.906395497243));
#50313=CARTESIAN_POINT('',(210.277543223595,-70.7420027758393,410.620680576218));
#50314=CARTESIAN_POINT('Origin',(211.655917770968,-72.0120072687899,408.906395497243));
#50315=CARTESIAN_POINT('Origin',(211.655917770968,-72.0119940563109,408.906387830743));
#50316=CARTESIAN_POINT('Origin',(208.730420887858,-72.0120072687899,406.554096622863));
#50317=CARTESIAN_POINT('',(220.926808850179,-70.742084448958,419.183439558327));
#50318=CARTESIAN_POINT('Ctrl Pts',(221.866228196796,-69.4720072829634,417.116184709025));
#50319=CARTESIAN_POINT('Ctrl Pts',(221.793911155898,-69.4720061785357,417.244522483259));
#50320=CARTESIAN_POINT('Ctrl Pts',(221.653554901702,-69.4970261445458,417.504572905438));
#50321=CARTESIAN_POINT('Ctrl Pts',(221.460643988658,-69.6083606205033,417.892354848133));
#50322=CARTESIAN_POINT('Ctrl Pts',(221.288915950418,-69.7913397669245,418.267516591053));
#50323=CARTESIAN_POINT('Ctrl Pts',(221.140717472848,-70.0432002703419,418.618591886083));
#50324=CARTESIAN_POINT('Ctrl Pts',(221.017898657018,-70.3602758159734,418.932833634663));
#50325=CARTESIAN_POINT('Ctrl Pts',(220.954019583338,-70.6094239199469,419.107063289083));
#50326=CARTESIAN_POINT('Ctrl Pts',(220.926793325828,-70.7420108908289,419.183399979823));
#50327=CARTESIAN_POINT('',(210.277557457508,-70.7420071496399,410.620695195203));
#50328=CARTESIAN_POINT('Ctrl Pts',(221.751276938898,-69.4654490974855,416.912272239873));
#50329=CARTESIAN_POINT('Ctrl Pts',(221.733129877708,-69.4642164587727,416.943814007983));
#50330=CARTESIAN_POINT('Ctrl Pts',(221.617992489818,-69.4612105224025,417.145906513633));
#50331=CARTESIAN_POINT('Ctrl Pts',(221.415156312278,-69.5133172277359,417.525769829863));
#50332=CARTESIAN_POINT('Ctrl Pts',(221.172069855068,-69.7138478877061,418.035004402343));
#50333=CARTESIAN_POINT('Ctrl Pts',(220.971244208648,-70.0353627268993,418.505648542643));
#50334=CARTESIAN_POINT('Ctrl Pts',(220.831492939438,-70.4245592719199,418.870035530053));
#50335=CARTESIAN_POINT('Ctrl Pts',(220.767019322678,-70.7132164602069,419.051296804093));
#50336=CARTESIAN_POINT('Ctrl Pts',(220.743986066728,-70.8407847846869,419.117507753173));
#50337=CARTESIAN_POINT('Ctrl Pts',(223.133361772338,-69.6040686792587,417.861603377653));
#50338=CARTESIAN_POINT('Ctrl Pts',(223.117828522468,-69.6011683474858,417.889594372033));
#50339=CARTESIAN_POINT('Ctrl Pts',(223.019091236198,-69.5865972268537,418.069323269803));
#50340=CARTESIAN_POINT('Ctrl Pts',(222.842402306488,-69.6065541544154,418.412681535193));
#50341=CARTESIAN_POINT('Ctrl Pts',(222.618697713768,-69.748647110422,418.894056406763));
#50342=CARTESIAN_POINT('Ctrl Pts',(222.418383540508,-70.0138432058709,419.363994557133));
#50343=CARTESIAN_POINT('Ctrl Pts',(222.265017884668,-70.3700332044191,419.749336964243));
#50344=CARTESIAN_POINT('Ctrl Pts',(222.188478557108,-70.653644403435,419.949352944663));
#50345=CARTESIAN_POINT('Ctrl Pts',(222.160509530328,-70.7819364497499,420.023365919093));
#50346=CARTESIAN_POINT('Ctrl Pts',(224.146167652288,-68.4191356321779,418.494670406743));
#50347=CARTESIAN_POINT('Ctrl Pts',(224.121229218938,-68.4143254993869,418.534145567303));
#50348=CARTESIAN_POINT('Ctrl Pts',(223.962191433298,-68.389321427153,418.787473307343));
#50349=CARTESIAN_POINT('Ctrl Pts',(223.671268120298,-68.4109449839659,419.270074399333));
#50350=CARTESIAN_POINT('Ctrl Pts',(223.288048525248,-68.6097419631932,419.947170649143));
#50351=CARTESIAN_POINT('Ctrl Pts',(222.931550755408,-68.9946417969064,420.611300967703));
#50352=CARTESIAN_POINT('Ctrl Pts',(222.649483805568,-69.5228226663634,421.159560115753));
#50353=CARTESIAN_POINT('Ctrl Pts',(222.505798556868,-69.9489645106603,421.445743086943));
#50354=CARTESIAN_POINT('Ctrl Pts',(222.452989851008,-70.142521288732,421.551828578973));
#50355=CARTESIAN_POINT('Ctrl Pts',(224.078317577708,-66.7429260460049,418.366818202673));
#50356=CARTESIAN_POINT('Ctrl Pts',(224.038561001198,-66.7373054148149,418.424746193413));
#50357=CARTESIAN_POINT('Ctrl Pts',(223.784876123258,-66.7103285449819,418.795940696103));
#50358=CARTESIAN_POINT('Ctrl Pts',(223.319573013478,-66.7662645270549,419.495730784653));
#50359=CARTESIAN_POINT('Ctrl Pts',(222.709982075748,-67.0970793500919,420.454658245053));
#50360=CARTESIAN_POINT('Ctrl Pts',(222.150306245338,-67.6936276079039,421.371481733313));
#50361=CARTESIAN_POINT('Ctrl Pts',(221.714848614868,-68.4779934089825,422.110189095833));
#50362=CARTESIAN_POINT('Ctrl Pts',(221.496099346358,-69.0941315197381,422.489429166423));
#50363=CARTESIAN_POINT('Ctrl Pts',(221.415994006008,-69.3716532420848,422.629330497173));
#50364=CARTESIAN_POINT('Origin',(219.548426388038,-69.4721780198135,420.897754057183));
#50365=CARTESIAN_POINT('Origin',(221.866229658128,-66.9320073823689,417.116182155053));
#50366=CARTESIAN_POINT('Origin',(263.115917770968,-66.93200726879,445.000000551893));
#50367=CARTESIAN_POINT('Origin',(235.232099333908,-66.9320072687899,403.750312439503));
#50368=CARTESIAN_POINT('Ctrl Pts',(237.233549882728,-70.8410255423379,402.628024620243));
#50369=CARTESIAN_POINT('Ctrl Pts',(237.166974214408,-70.7127222484639,402.651184041943));
#50370=CARTESIAN_POINT('Ctrl Pts',(236.984869388708,-70.4229586079244,402.715961802783));
#50371=CARTESIAN_POINT('Ctrl Pts',(236.618402976028,-70.0324228883722,402.856575913253));
#50372=CARTESIAN_POINT('Ctrl Pts',(236.146471696558,-69.711449747235,403.058146362133));
#50373=CARTESIAN_POINT('Ctrl Pts',(235.638095324218,-69.512638144513,403.301110138693));
#50374=CARTESIAN_POINT('Ctrl Pts',(235.260489121208,-69.4612407849914,403.502837229903));
#50375=CARTESIAN_POINT('Ctrl Pts',(235.059875954418,-69.4642146335529,403.617129368273));
#50376=CARTESIAN_POINT('Ctrl Pts',(235.028428642488,-69.4654396674749,403.635221145173));
#50377=CARTESIAN_POINT('Ctrl Pts',(238.139422700518,-70.7821785594619,404.044539750673));
#50378=CARTESIAN_POINT('Ctrl Pts',(238.065000599578,-70.6531438863329,404.072662858133));
#50379=CARTESIAN_POINT('Ctrl Pts',(237.864062326518,-70.3684786785249,404.149556582403));
#50380=CARTESIAN_POINT('Ctrl Pts',(237.476623171508,-70.0112367740756,404.303798588993));
#50381=CARTESIAN_POINT('Ctrl Pts',(237.005646976138,-69.7468008290302,404.504691162843));
#50382=CARTESIAN_POINT('Ctrl Pts',(236.525331980678,-69.6062166524363,404.728125988013));
#50383=CARTESIAN_POINT('Ctrl Pts',(236.184054767208,-69.5867023581791,404.903827170923));
#50384=CARTESIAN_POINT('Ctrl Pts',(236.005640525168,-69.6011587121201,405.001840027323));
#50385=CARTESIAN_POINT('Ctrl Pts',(235.977733092948,-69.6040471487245,405.017326135553));
#50386=CARTESIAN_POINT('Ctrl Pts',(239.667946446748,-70.1428862842576,404.336973689953));
#50387=CARTESIAN_POINT('Ctrl Pts',(239.561274231638,-69.9482081499974,404.390073749173));
#50388=CARTESIAN_POINT('Ctrl Pts',(239.273773460878,-69.5204913988231,404.534422144333));
#50389=CARTESIAN_POINT('Ctrl Pts',(238.722549836198,-68.9908005466803,404.818062860253));
#50390=CARTESIAN_POINT('Ctrl Pts',(238.056991236348,-68.6071038509312,405.175476844673));
#50391=CARTESIAN_POINT('Ctrl Pts',(237.381404445628,-68.4105256300779,405.558075870093));
#50392=CARTESIAN_POINT('Ctrl Pts',(236.901719399648,-68.3894990752359,405.847325697563));
#50393=CARTESIAN_POINT('Ctrl Pts',(236.650244885598,-68.4143084253989,406.005197780233));
#50394=CARTESIAN_POINT('Ctrl Pts',(236.610887702388,-68.4190995018019,406.030060962223));
#50395=CARTESIAN_POINT('Ctrl Pts',(240.745512611478,-69.3721764983919,403.299925922353));
#50396=CARTESIAN_POINT('Ctrl Pts',(240.604838520268,-69.0930496471821,403.380472822573));
#50397=CARTESIAN_POINT('Ctrl Pts',(240.223846195178,-68.4746082940245,403.600235607753));
#50398=CARTESIAN_POINT('Ctrl Pts',(239.481065738028,-67.6878508746749,404.038158442043));
#50399=CARTESIAN_POINT('Ctrl Pts',(238.562058543708,-67.0928621596819,404.599355204583));
#50400=CARTESIAN_POINT('Ctrl Pts',(237.605022300298,-66.7653976675589,405.208017414293));
#50401=CARTESIAN_POINT('Ctrl Pts',(236.909407855438,-66.7105257118319,405.670635844973));
#50402=CARTESIAN_POINT('Ctrl Pts',(236.540930137708,-66.7372867844729,405.922461582133));
#50403=CARTESIAN_POINT('Ctrl Pts',(236.483175678898,-66.7428833566679,405.962098286683));
#50404=CARTESIAN_POINT('',(237.299337446915,-70.7420402776057,402.810888231475));
#50405=CARTESIAN_POINT('Origin',(239.013670773968,-69.4721762071727,401.432509576753));
#50406=CARTESIAN_POINT('Ctrl Pts',(237.299306020227,-70.7420200455038,402.810887527682));
#50407=CARTESIAN_POINT('Ctrl Pts',(237.243212043783,-70.6445951393941,402.830894421642));
#50408=CARTESIAN_POINT('Ctrl Pts',(237.181240654867,-70.5513567221656,402.853463025695));
#50409=CARTESIAN_POINT('Ctrl Pts',(237.089965079941,-70.4311536188862,402.887559389488));
#50410=CARTESIAN_POINT('Ctrl Pts',(237.065170544958,-70.4000028232924,402.896896373708));
#50411=CARTESIAN_POINT('Ctrl Pts',(236.943547013715,-70.2540727483776,402.943096611271));
#50412=CARTESIAN_POINT('Ctrl Pts',(236.838285008499,-70.147886017895,402.984237043943));
#50413=CARTESIAN_POINT('Ctrl Pts',(236.721167126839,-70.047920025344,403.031965775962));
#50414=CARTESIAN_POINT('Ctrl Pts',(236.715633996361,-70.0432370796357,403.034224934696));
#50415=CARTESIAN_POINT('Ctrl Pts',(236.603413091615,-69.9490612742504,403.080131984757));
#50416=CARTESIAN_POINT('Ctrl Pts',(236.491135927334,-69.8694544987991,403.12766427235));
#50417=CARTESIAN_POINT('Ctrl Pts',(236.331150141304,-69.7740400952014,403.198202289507));
#50418=CARTESIAN_POINT('Ctrl Pts',(236.286358613182,-69.7491804686927,403.21823503636));
#50419=CARTESIAN_POINT('Ctrl Pts',(236.16218220769,-69.6852131557635,403.274625319477));
#50420=CARTESIAN_POINT('Ctrl Pts',(236.081996177396,-69.6493657107355,403.311979884422));
#50421=CARTESIAN_POINT('Ctrl Pts',(235.915390721252,-69.5855318937611,403.391686852879));
#50422=CARTESIAN_POINT('Ctrl Pts',(235.828898456121,-69.5581670824827,403.434204879921));
#50423=CARTESIAN_POINT('Ctrl Pts',(235.700509048139,-69.5258783396488,403.499122783802));
#50424=CARTESIAN_POINT('Ctrl Pts',(235.658852883162,-69.5166925224,403.520464743105));
#50425=CARTESIAN_POINT('Ctrl Pts',(235.488419035691,-69.4843334129535,403.608922427488));
#50426=CARTESIAN_POINT('Ctrl Pts',(235.359324546871,-69.4720048208222,403.678623129688));
#50427=CARTESIAN_POINT('Ctrl Pts',(235.23210195903,-69.4720073298541,403.75031096033));
#50428=CARTESIAN_POINT('Origin',(312.119295247928,-72.0120072687901,499.373047478893));
#50429=CARTESIAN_POINT('',(228.736597916929,-70.7420026857022,392.161625909054));
#50430=CARTESIAN_POINT('',(237.299318413618,-70.7420108634959,402.810877563033));
#50431=CARTESIAN_POINT('Origin',(227.022312716318,-72.0120072687899,393.540000551893));
#50432=CARTESIAN_POINT('Origin',(227.022312716318,-72.0120072687899,393.540000551893));
#50433=CARTESIAN_POINT('Origin',(227.022305049898,-72.0119940551319,393.540000551893));
#50434=CARTESIAN_POINT('Ctrl Pts',(225.638731539658,-72.7677512569999,391.539590768683));
#50435=CARTESIAN_POINT('Ctrl Pts',(225.701233575478,-72.8415267130749,391.532135400383));
#50436=CARTESIAN_POINT('Ctrl Pts',(226.003100564118,-73.1792881921419,391.496357986363));
#50437=CARTESIAN_POINT('Ctrl Pts',(226.618188529078,-73.7177818201399,391.426026824253));
#50438=CARTESIAN_POINT('Ctrl Pts',(227.544153998748,-74.2773859034239,391.328484143693));
#50439=CARTESIAN_POINT('Ctrl Pts',(228.602549223918,-74.6941844569289,391.229364067463));
#50440=CARTESIAN_POINT('Ctrl Pts',(229.794873524898,-74.9488215698489,391.135288067703));
#50441=CARTESIAN_POINT('Ctrl Pts',(231.115092556868,-75.0078404229169,391.055676779643));
#50442=CARTESIAN_POINT('Ctrl Pts',(232.135101469358,-74.8793277233339,391.018196529693));
#50443=CARTESIAN_POINT('Ctrl Pts',(232.708118783838,-74.7445966300439,391.007075109083));
#50444=CARTESIAN_POINT('Ctrl Pts',(232.827528105778,-74.7136854275459,391.005217023583));
#50445=CARTESIAN_POINT('Ctrl Pts',(226.729205733288,-72.0150401412129,390.502814873693));
#50446=CARTESIAN_POINT('Ctrl Pts',(226.784485182628,-72.0696574342109,390.501671320983));
#50447=CARTESIAN_POINT('Ctrl Pts',(227.051133216628,-72.3183990485599,390.496604468393));
#50448=CARTESIAN_POINT('Ctrl Pts',(227.591135925408,-72.7034694767339,390.491103408133));
#50449=CARTESIAN_POINT('Ctrl Pts',(228.394849203928,-73.0785538001049,390.497473302493));
#50450=CARTESIAN_POINT('Ctrl Pts',(229.301912439038,-73.3269041512489,390.525172264273));
#50451=CARTESIAN_POINT('Ctrl Pts',(230.309431538478,-73.4353515823529,390.584022187893));
#50452=CARTESIAN_POINT('Ctrl Pts',(231.407183411688,-73.3818065903929,390.686408043543));
#50453=CARTESIAN_POINT('Ctrl Pts',(232.239274844198,-73.2090456373969,390.801031497173));
#50454=CARTESIAN_POINT('Ctrl Pts',(232.700255290318,-73.0666989540409,390.880006490083));
#50455=CARTESIAN_POINT('Ctrl Pts',(232.796017495648,-73.0350067849759,390.897138866913));
#50456=CARTESIAN_POINT('Ctrl Pts',(228.085997126648,-71.0785068454429,390.838423841053));
#50457=CARTESIAN_POINT('Ctrl Pts',(228.125915950258,-71.1136849925869,390.845133249633));
#50458=CARTESIAN_POINT('Ctrl Pts',(228.318823985898,-71.2742945628339,390.878024909003));
#50459=CARTESIAN_POINT('Ctrl Pts',(228.712998825878,-71.5264525149989,390.950035883993));
#50460=CARTESIAN_POINT('Ctrl Pts',(229.309457181038,-71.7799841162819,391.072990587163));
#50461=CARTESIAN_POINT('Ctrl Pts',(229.995069125098,-71.9582914907429,391.232931398903));
#50462=CARTESIAN_POINT('Ctrl Pts',(230.772193181038,-72.0525390598589,391.438419215633));
#50463=CARTESIAN_POINT('Ctrl Pts',(231.638597324058,-72.0476828902759,391.699013951043));
#50464=CARTESIAN_POINT('Ctrl Pts',(232.313310257318,-71.9600636709789,391.931215466993));
#50465=CARTESIAN_POINT('Ctrl Pts',(232.694495845898,-71.8813627885119,392.074251652513));
#50466=CARTESIAN_POINT('Ctrl Pts',(232.774029563598,-71.8636344410639,392.104641802563));
#50467=CARTESIAN_POINT('Ctrl Pts',(228.756126450238,-70.6159509551309,392.310693601373));
#50468=CARTESIAN_POINT('Ctrl Pts',(228.783335561338,-70.6450625854709,392.321281376383));
#50469=CARTESIAN_POINT('Ctrl Pts',(228.915775844658,-70.7803298660319,392.372718306873));
#50470=CARTESIAN_POINT('Ctrl Pts',(229.195806365828,-71.0134407518539,392.480480568223));
#50471=CARTESIAN_POINT('Ctrl Pts',(229.645578187428,-71.2937625231659,392.650805808573));
#50472=CARTESIAN_POINT('Ctrl Pts',(230.195161865718,-71.5496287328339,392.855527628773));
#50473=CARTESIAN_POINT('Ctrl Pts',(230.858125249808,-71.7716399183579,393.098370203183));
#50474=CARTESIAN_POINT('Ctrl Pts',(231.646794450178,-71.9425273223459,393.382263252623));
#50475=CARTESIAN_POINT('Ctrl Pts',(232.305206926388,-72.0096382157559,393.614933045543));
#50476=CARTESIAN_POINT('Ctrl Pts',(232.694885752718,-72.0211411690119,393.751000084983));
#50477=CARTESIAN_POINT('Ctrl Pts',(232.777008130648,-72.0223135621609,393.779603362203));
#50478=CARTESIAN_POINT('Ctrl Pts',(228.736612778339,-70.7420068809478,392.161639950096));
#50479=CARTESIAN_POINT('Ctrl Pts',(228.74403795138,-70.7492044424187,392.164243359666));
#50480=CARTESIAN_POINT('Ctrl Pts',(228.751537755498,-70.7563928376238,392.166872853459));
#50481=CARTESIAN_POINT('Ctrl Pts',(228.759112290133,-70.763571339069,392.169528479623));
#50482=CARTESIAN_POINT('Ctrl Pts',(228.809211693663,-70.8110513042359,392.187093292937));
#50483=CARTESIAN_POINT('Ctrl Pts',(228.862583719871,-70.8580999963968,392.205802451487));
#50484=CARTESIAN_POINT('Ctrl Pts',(228.919273539135,-70.9045511124965,392.225676018046));
#50485=CARTESIAN_POINT('Ctrl Pts',(228.962724221884,-70.9401542019974,392.240908383343));
#50486=CARTESIAN_POINT('Ctrl Pts',(229.008123316606,-70.9754058614114,392.256824573291));
#50487=CARTESIAN_POINT('Ctrl Pts',(229.055472831776,-71.0102232739626,392.273427482023));
#50488=CARTESIAN_POINT('Ctrl Pts',(229.080041424926,-71.0282892423348,392.282042356078));
#50489=CARTESIAN_POINT('Ctrl Pts',(229.105137428495,-71.0462403635194,392.29084252611));
#50490=CARTESIAN_POINT('Ctrl Pts',(229.130755854209,-71.0640622097133,392.299825985934));
#50491=CARTESIAN_POINT('Ctrl Pts',(229.193064119902,-71.1074078992641,392.321675252076));
#50492=CARTESIAN_POINT('Ctrl Pts',(229.258465836879,-71.14998880754,392.344609885107));
#50493=CARTESIAN_POINT('Ctrl Pts',(229.326918348435,-71.1916308944421,392.368610806374));
#50494=CARTESIAN_POINT('Ctrl Pts',(229.36603060828,-71.2154242671967,392.382324405011));
#50495=CARTESIAN_POINT('Ctrl Pts',(229.40613801284,-71.2389111258167,392.396385806151));
#50496=CARTESIAN_POINT('Ctrl Pts',(229.447225366973,-71.2620589077046,392.410788824469));
#50497=CARTESIAN_POINT('Ctrl Pts',(229.494799950007,-71.288861462766,392.427465916615));
#50498=CARTESIAN_POINT('Ctrl Pts',(229.543696252613,-71.3152111239886,392.444609773287));
#50499=CARTESIAN_POINT('Ctrl Pts',(229.59395706903,-71.3410926562254,392.462233906472));
#50500=CARTESIAN_POINT('Ctrl Pts',(229.670815547899,-71.38067050912,392.489184604145));
#50501=CARTESIAN_POINT('Ctrl Pts',(229.750864959679,-71.4191559802305,392.517258475578));
#50502=CARTESIAN_POINT('Ctrl Pts',(229.834329102691,-71.4564687983865,392.54652792326));
#50503=CARTESIAN_POINT('Ctrl Pts',(229.859841020467,-71.4678739541152,392.555474516559));
#50504=CARTESIAN_POINT('Ctrl Pts',(229.885671907711,-71.4791691936545,392.564532782266));
#50505=CARTESIAN_POINT('Ctrl Pts',(229.911827890448,-71.4903512773118,392.573704679131));
#50506=CARTESIAN_POINT('Ctrl Pts',(229.988742853775,-71.5232336034354,392.600675797678));
#50507=CARTESIAN_POINT('Ctrl Pts',(230.068471344098,-71.5551392419008,392.628634979833));
#50508=CARTESIAN_POINT('Ctrl Pts',(230.151226023293,-71.5859845480201,392.657655092177));
#50509=CARTESIAN_POINT('Ctrl Pts',(230.234662022126,-71.6170838036803,392.686914127233));
#50510=CARTESIAN_POINT('Ctrl Pts',(230.321173870445,-71.6471054203405,392.717251501234));
#50511=CARTESIAN_POINT('Ctrl Pts',(230.411024902909,-71.6759139021873,392.748757605007));
#50512=CARTESIAN_POINT('Ctrl Pts',(230.426345128825,-71.6808259486944,392.754129614814));
#50513=CARTESIAN_POINT('Ctrl Pts',(230.441762397531,-71.6857026097513,392.75953558958));
#50514=CARTESIAN_POINT('Ctrl Pts',(230.457277962987,-71.6905430691913,392.76497595883));
#50515=CARTESIAN_POINT('Ctrl Pts',(230.545245222552,-71.7179866034395,392.79582074984));
#50516=CARTESIAN_POINT('Ctrl Pts',(230.63636403198,-71.7442659054211,392.827769177735));
#50517=CARTESIAN_POINT('Ctrl Pts',(230.730813923741,-71.7691988042511,392.860887773716));
#50518=CARTESIAN_POINT('Ctrl Pts',(230.760044347557,-71.7769150566064,392.871137341806));
#50519=CARTESIAN_POINT('Ctrl Pts',(230.789593588474,-71.7845020756735,392.881498908917));
#50520=CARTESIAN_POINT('Ctrl Pts',(230.819466283583,-71.7919537134946,392.891974213097));
#50521=CARTESIAN_POINT('Ctrl Pts',(230.908976721051,-71.8142817745812,392.923362377314));
#50522=CARTESIAN_POINT('Ctrl Pts',(231.001392860546,-71.8353967743901,392.955772267799));
#50523=CARTESIAN_POINT('Ctrl Pts',(231.096866864063,-71.8551008150376,392.989260375604));
#50524=CARTESIAN_POINT('Ctrl Pts',(231.190683495745,-71.8744628052754,393.022167149802));
#50525=CARTESIAN_POINT('Ctrl Pts',(231.287442455986,-71.8924577821863,393.056101914368));
#50526=CARTESIAN_POINT('Ctrl Pts',(231.386931110687,-71.9088265655427,393.090990503202));
#50527=CARTESIAN_POINT('Ctrl Pts',(231.461377080757,-71.9210750973928,393.117097146698));
#50528=CARTESIAN_POINT('Ctrl Pts',(231.537350586221,-71.9324134528414,393.143737550279));
#50529=CARTESIAN_POINT('Ctrl Pts',(231.61474610887,-71.9427410029754,393.170874910618));
#50530=CARTESIAN_POINT('Ctrl Pts',(231.687812320525,-71.9524908559145,393.196494275234));
#50531=CARTESIAN_POINT('Ctrl Pts',(231.762145631757,-71.9613399669065,393.222556457012));
#50532=CARTESIAN_POINT('Ctrl Pts',(231.837658155136,-71.9692011295691,393.249030825801));
#50533=CARTESIAN_POINT('Ctrl Pts',(231.948168690718,-71.9807057285055,393.287775348473));
#50534=CARTESIAN_POINT('Ctrl Pts',(232.061196287319,-71.9900966506596,393.327401492746));
#50535=CARTESIAN_POINT('Ctrl Pts',(232.176755960482,-71.9971271824967,393.367917803244));
#50536=CARTESIAN_POINT('Ctrl Pts',(232.292315633645,-72.0041577143338,393.408434113742));
#50537=CARTESIAN_POINT('Ctrl Pts',(232.410407981347,-72.0088279534613,393.449840809688));
#50538=CARTESIAN_POINT('Ctrl Pts',(232.531007414461,-72.0108586572646,393.492132222973));
#50539=CARTESIAN_POINT('Ctrl Pts',(232.576155932945,-72.0116188869426,393.507964757215));
#50540=CARTESIAN_POINT('Ctrl Pts',(232.621655364709,-72.0120088644348,393.523921124644));
#50541=CARTESIAN_POINT('Ctrl Pts',(232.667503020154,-72.0120105964114,393.540000551869));
#50542=CARTESIAN_POINT('Origin',(232.667503020198,-74.5520072687899,393.540000551893));
#50543=CARTESIAN_POINT('Origin',(220.367523674428,-74.5520072687899,393.540000551893));
#50544=CARTESIAN_POINT('Origin',(317.572435894888,-69.4720072687901,499.134199992603));
#50545=CARTESIAN_POINT('Origin',(239.013637433378,-69.4720072687899,401.432533532013));
#50546=CARTESIAN_POINT('Origin',(239.013637433378,-69.4720072687899,401.432533532013));
#50547=CARTESIAN_POINT('Origin',(219.548450751088,-69.47200726879,420.897720214303));
#50548=CARTESIAN_POINT('Origin',(219.548450751088,-69.47200726879,420.897720214303));
#50549=CARTESIAN_POINT('Origin',(219.548450751088,-69.47200726879,420.897720214303));
#50550=CARTESIAN_POINT('Origin',(207.104559699488,-69.4720072687899,410.891983724703));
#50551=CARTESIAN_POINT('Ctrl Pts',(211.655917770968,-72.0120072687899,414.551585801243));
#50552=CARTESIAN_POINT('Ctrl Pts',(211.615573220631,-72.0120072687893,414.436550636498));
#50553=CARTESIAN_POINT('Ctrl Pts',(211.57601762646,-72.0095636111052,414.323713264967));
#50554=CARTESIAN_POINT('Ctrl Pts',(211.537236944843,-72.004934580418,414.213102620862));
#50555=CARTESIAN_POINT('Ctrl Pts',(211.497128231632,-72.0001470301086,414.098704151893));
#50556=CARTESIAN_POINT('Ctrl Pts',(211.457848731293,-71.9930221141195,413.986687132813));
#50557=CARTESIAN_POINT('Ctrl Pts',(211.41940551576,-71.9838027053749,413.877055455955));
#50558=CARTESIAN_POINT('Ctrl Pts',(211.401061356736,-71.979403429774,413.824741910211));
#50559=CARTESIAN_POINT('Ctrl Pts',(211.382907910837,-71.9745266060013,413.772971132622));
#50560=CARTESIAN_POINT('Ctrl Pts',(211.364947347806,-71.9691951485483,413.721741803245));
#50561=CARTESIAN_POINT('Ctrl Pts',(211.323470638976,-71.9568831008668,413.603436827254));
#50562=CARTESIAN_POINT('Ctrl Pts',(211.283018364773,-71.9421444368132,413.488024602253));
#50563=CARTESIAN_POINT('Ctrl Pts',(211.2436852705,-71.9253093502899,413.375850557814));
#50564=CARTESIAN_POINT('Ctrl Pts',(211.203770283176,-71.9082252058153,413.262017012686));
#50565=CARTESIAN_POINT('Ctrl Pts',(211.165007777648,-71.8889826584265,413.151518239305));
#50566=CARTESIAN_POINT('Ctrl Pts',(211.127528730766,-71.8679429935169,413.044675473092));
#50567=CARTESIAN_POINT('Ctrl Pts',(211.120025920614,-71.8637311304994,413.023286962504));
#50568=CARTESIAN_POINT('Ctrl Pts',(211.112574647037,-71.8594472855253,413.002044838281));
#50569=CARTESIAN_POINT('Ctrl Pts',(211.105176113533,-71.8550944057301,412.980951487548));
#50570=CARTESIAN_POINT('Ctrl Pts',(211.069370613624,-71.8340284692115,412.878869369868));
#50571=CARTESIAN_POINT('Ctrl Pts',(211.034798364851,-71.811350446314,412.780274163183));
#50572=CARTESIAN_POINT('Ctrl Pts',(211.001389235961,-71.7872977520792,412.684998500664));
#50573=CARTESIAN_POINT('Ctrl Pts',(210.966916846553,-71.7624795700572,412.586690647433));
#50574=CARTESIAN_POINT('Ctrl Pts',(210.933683122997,-71.7361978239172,412.491916576845));
#50575=CARTESIAN_POINT('Ctrl Pts',(210.901620789353,-71.7086604136442,412.400480282124));
#50576=CARTESIAN_POINT('Ctrl Pts',(210.894655929852,-71.7026784974274,412.380617693421));
#50577=CARTESIAN_POINT('Ctrl Pts',(210.887746371089,-71.6966371365098,412.360912577864));
#50578=CARTESIAN_POINT('Ctrl Pts',(210.880891458605,-71.6905381476994,412.34136288252));
#50579=CARTESIAN_POINT('Ctrl Pts',(210.848995685452,-71.6621596725513,412.250398534045));
#50580=CARTESIAN_POINT('Ctrl Pts',(210.818278555373,-71.6325417447364,412.162804616693));
#50581=CARTESIAN_POINT('Ctrl Pts',(210.788658026324,-71.6018271779366,412.078337223404));
#50582=CARTESIAN_POINT('Ctrl Pts',(210.758237710562,-71.5702832842081,411.991589118024));
#50583=CARTESIAN_POINT('Ctrl Pts',(210.728974349512,-71.5375825443219,411.908138238221));
#50584=CARTESIAN_POINT('Ctrl Pts',(210.700775922478,-71.5038254269898,411.827724301354));
#50585=CARTESIAN_POINT('Ctrl Pts',(210.697038832652,-71.4993516533435,411.817067178353));
#50586=CARTESIAN_POINT('Ctrl Pts',(210.693320438431,-71.494859252256,411.806463406203));
#50587=CARTESIAN_POINT('Ctrl Pts',(210.689620516852,-71.490348391484,411.795912389948));
#50588=CARTESIAN_POINT('Ctrl Pts',(210.658860846593,-71.4528468966634,411.708195454875));
#50589=CARTESIAN_POINT('Ctrl Pts',(210.629375375526,-71.4140777951987,411.624127971558));
#50590=CARTESIAN_POINT('Ctrl Pts',(210.601096592513,-71.3741434341638,411.543485356505));
#50591=CARTESIAN_POINT('Ctrl Pts',(210.575316107032,-71.3377370861809,411.469967137362));
#50592=CARTESIAN_POINT('Ctrl Pts',(210.550538616785,-71.3003613442115,411.399295251388));
#50593=CARTESIAN_POINT('Ctrl Pts',(210.526705473455,-71.2620580055459,411.331308856496));
#50594=CARTESIAN_POINT('Ctrl Pts',(210.494241662258,-71.2098839243747,411.238702629227));
#50595=CARTESIAN_POINT('Ctrl Pts',(210.463524675797,-71.1559856697735,411.151085654466));
#50596=CARTESIAN_POINT('Ctrl Pts',(210.434593550148,-71.1007413437056,411.068585459237));
#50597=CARTESIAN_POINT('Ctrl Pts',(210.418987135777,-71.0709407111722,411.024082101572));
#50598=CARTESIAN_POINT('Ctrl Pts',(210.403900955729,-71.0407484329972,410.981066958717));
#50599=CARTESIAN_POINT('Ctrl Pts',(210.389345073945,-71.0102237227438,410.939555152717));
#50600=CARTESIAN_POINT('Ctrl Pts',(210.360835380456,-70.9504368856354,410.858248579687));
#50601=CARTESIAN_POINT('Ctrl Pts',(210.334359040546,-70.8893746647691,410.782710452317));
#50602=CARTESIAN_POINT('Ctrl Pts',(210.309876500781,-70.8274387235966,410.712877624817));
#50603=CARTESIAN_POINT('Ctrl Pts',(210.298687198858,-70.7991320220723,410.680961794248));
#50604=CARTESIAN_POINT('Ctrl Pts',(210.28791478507,-70.7706425611211,410.650237145439));
#50605=CARTESIAN_POINT('Ctrl Pts',(210.277557554618,-70.7420072391133,410.62069507443));
#50606=CARTESIAN_POINT('Ctrl Pts',(209.121123721488,-74.7135102960079,414.712287298723));
#50607=CARTESIAN_POINT('Ctrl Pts',(209.122983464708,-74.7444894757819,414.592657233853));
#50608=CARTESIAN_POINT('Ctrl Pts',(209.134105034848,-74.8792977192369,414.019422444493));
#50609=CARTESIAN_POINT('Ctrl Pts',(209.171593985388,-75.0078404201239,412.999175337183));
#50610=CARTESIAN_POINT('Ctrl Pts',(209.251205289358,-74.9488215699039,411.678956306283));
#50611=CARTESIAN_POINT('Ctrl Pts',(209.345281286278,-74.6941844563889,410.486632004503));
#50612=CARTESIAN_POINT('Ctrl Pts',(209.444401360718,-74.2773859031249,409.428236781593));
#50613=CARTESIAN_POINT('Ctrl Pts',(209.541944049408,-73.7177818197019,408.502271304853));
#50614=CARTESIAN_POINT('Ctrl Pts',(209.612256946988,-73.1794278704339,407.887342904063));
#50615=CARTESIAN_POINT('Ctrl Pts',(209.648018171018,-72.8418519885089,407.585607074523));
#50616=CARTESIAN_POINT('Ctrl Pts',(209.655457208818,-72.7682536630759,407.523240000553));
#50617=CARTESIAN_POINT('Ctrl Pts',(209.013153141798,-73.0348272383849,414.680642732713));
#50618=CARTESIAN_POINT('Ctrl Pts',(208.995986491448,-73.0665857466229,414.584704646173));
#50619=CARTESIAN_POINT('Ctrl Pts',(208.916975523978,-73.2090053014829,414.123551936943));
#50620=CARTESIAN_POINT('Ctrl Pts',(208.802325249018,-73.3818065876669,413.291266191913));
#50621=CARTESIAN_POINT('Ctrl Pts',(208.699939410138,-73.4353515827459,412.193514319793));
#50622=CARTESIAN_POINT('Ctrl Pts',(208.641089483568,-73.3269041507879,411.185995219493));
#50623=CARTESIAN_POINT('Ctrl Pts',(208.613390519918,-73.0785538002929,410.278931986753));
#50624=CARTESIAN_POINT('Ctrl Pts',(208.607020634118,-72.7034694752909,409.475218700813));
#50625=CARTESIAN_POINT('Ctrl Pts',(208.612520244838,-72.3184989335639,408.935356080983));
#50626=CARTESIAN_POINT('Ctrl Pts',(208.617583669858,-72.0698969776509,408.668824761813));
#50627=CARTESIAN_POINT('Ctrl Pts',(208.618724302488,-72.0154120774029,408.613665002433));
#50628=CARTESIAN_POINT('Ctrl Pts',(210.220731177198,-71.8635340023709,414.658562876293));
#50629=CARTESIAN_POINT('Ctrl Pts',(210.190282605478,-71.8813001977719,414.578881749843));
#50630=CARTESIAN_POINT('Ctrl Pts',(210.047186932298,-71.9600432143439,414.197550598173));
#50631=CARTESIAN_POINT('Ctrl Pts',(209.814931162538,-72.0476828890719,413.522680104543));
#50632=CARTESIAN_POINT('Ctrl Pts',(209.554336436448,-72.0525390603359,412.656275962093));
#50633=CARTESIAN_POINT('Ctrl Pts',(209.348848618108,-71.9582914907669,411.879151905633));
#50634=CARTESIAN_POINT('Ctrl Pts',(209.188907805368,-71.7799841165459,411.193539962853));
#50635=CARTESIAN_POINT('Ctrl Pts',(209.065953106938,-71.5264525146379,410.597081603543));
#50636=CARTESIAN_POINT('Ctrl Pts',(208.993960798188,-71.2743599704639,410.203009018083));
#50637=CARTESIAN_POINT('Ctrl Pts',(208.961082152008,-71.1138396640759,410.010184514773));
#50638=CARTESIAN_POINT('Ctrl Pts',(208.954386755368,-71.0787464051469,409.970351781083));
#50639=CARTESIAN_POINT('Ctrl Pts',(211.895682611298,-72.0223201904569,414.661556116033));
#50640=CARTESIAN_POINT('Ctrl Pts',(211.867025508458,-72.0211503125039,414.579278414173));
#50641=CARTESIAN_POINT('Ctrl Pts',(211.730904594288,-72.0096538864489,414.189443459553));
#50642=CARTESIAN_POINT('Ctrl Pts',(211.498180472458,-71.9425273227339,413.530877231143));
#50643=CARTESIAN_POINT('Ctrl Pts',(211.214287421758,-71.7716399182749,412.742208030703));
#50644=CARTESIAN_POINT('Ctrl Pts',(210.971444847568,-71.5496287330819,412.079244646653));
#50645=CARTESIAN_POINT('Ctrl Pts',(210.766723027528,-71.2937625227309,411.529660968183));
#50646=CARTESIAN_POINT('Ctrl Pts',(210.596397786528,-71.0134407536249,411.079889147063));
#50647=CARTESIAN_POINT('Ctrl Pts',(210.488663479068,-70.7803903280709,410.799931260843));
#50648=CARTESIAN_POINT('Ctrl Pts',(210.437248133258,-70.6451928569439,410.667545895773));
#50649=CARTESIAN_POINT('Ctrl Pts',(210.426682931138,-70.6161492097429,410.640394546293));
#50650=CARTESIAN_POINT('Origin',(211.655917770968,-74.5520139244089,414.551585800783));
#50651=CARTESIAN_POINT('Origin',(211.655917770968,-74.55200726879,487.748394648433));
#50652=CARTESIAN_POINT('Origin',(211.655917770968,-74.55200726879,475.448415302663));
#50653=CARTESIAN_POINT('Ctrl Pts',(209.655507987758,-72.767751257,482.477186783203));
#50654=CARTESIAN_POINT('Ctrl Pts',(209.648052619458,-72.841526713075,482.414684747383));
#50655=CARTESIAN_POINT('Ctrl Pts',(209.612275205438,-73.179288192142,482.112817758743));
#50656=CARTESIAN_POINT('Ctrl Pts',(209.541944043328,-73.71778182014,481.497729793783));
#50657=CARTESIAN_POINT('Ctrl Pts',(209.444401362768,-74.277385903423,480.571764324113));
#50658=CARTESIAN_POINT('Ctrl Pts',(209.345281286538,-74.694184456929,479.513369098943));
#50659=CARTESIAN_POINT('Ctrl Pts',(209.251205286778,-74.948821569849,478.321044797963));
#50660=CARTESIAN_POINT('Ctrl Pts',(209.171593998718,-75.007840422917,477.000825765993));
#50661=CARTESIAN_POINT('Ctrl Pts',(209.134113748768,-74.879327723334,475.980816853503));
#50662=CARTESIAN_POINT('Ctrl Pts',(209.122992328158,-74.744596630044,475.407799539023));
#50663=CARTESIAN_POINT('Ctrl Pts',(209.121134242658,-74.713685427546,475.288390217083));
#50664=CARTESIAN_POINT('Ctrl Pts',(208.618732092768,-72.015040141213,481.386712589573));
#50665=CARTESIAN_POINT('Ctrl Pts',(208.617588540058,-72.069657434211,481.331433140233));
#50666=CARTESIAN_POINT('Ctrl Pts',(208.612521687468,-72.31839904856,481.064785106233));
#50667=CARTESIAN_POINT('Ctrl Pts',(208.607020627208,-72.703469476734,480.524782397453));
#50668=CARTESIAN_POINT('Ctrl Pts',(208.613390521568,-73.078553800105,479.721069118933));
#50669=CARTESIAN_POINT('Ctrl Pts',(208.641089483348,-73.326904151249,478.814005883823));
#50670=CARTESIAN_POINT('Ctrl Pts',(208.699939406968,-73.435351582353,477.806486784383));
#50671=CARTESIAN_POINT('Ctrl Pts',(208.802325262618,-73.381806590393,476.708734911173));
#50672=CARTESIAN_POINT('Ctrl Pts',(208.916948716248,-73.209045637397,475.876643478663));
#50673=CARTESIAN_POINT('Ctrl Pts',(208.995923709158,-73.066698954042,475.415663032543));
#50674=CARTESIAN_POINT('Ctrl Pts',(209.013056085988,-73.035006784976,475.319900827213));
#50675=CARTESIAN_POINT('Ctrl Pts',(208.954341060128,-71.078506845443,480.029921196213));
#50676=CARTESIAN_POINT('Ctrl Pts',(208.961050468708,-71.113684992587,479.990002372603));
#50677=CARTESIAN_POINT('Ctrl Pts',(208.993942128078,-71.274294562834,479.797094336963));
#50678=CARTESIAN_POINT('Ctrl Pts',(209.065953103068,-71.526452514999,479.402919496983));
#50679=CARTESIAN_POINT('Ctrl Pts',(209.188907806238,-71.779984116282,478.806461141823));
#50680=CARTESIAN_POINT('Ctrl Pts',(209.348848617978,-71.958291490743,478.120849197763));
#50681=CARTESIAN_POINT('Ctrl Pts',(209.554336434708,-72.052539059859,477.343725141823));
#50682=CARTESIAN_POINT('Ctrl Pts',(209.814931170118,-72.047682890276,476.477320998803));
#50683=CARTESIAN_POINT('Ctrl Pts',(210.047132686068,-71.960063670979,475.802608065543));
#50684=CARTESIAN_POINT('Ctrl Pts',(210.190168871588,-71.881362788512,475.421422476963));
#50685=CARTESIAN_POINT('Ctrl Pts',(210.220559021638,-71.863634441064,475.341888759263));
#50686=CARTESIAN_POINT('Ctrl Pts',(210.426610820448,-70.615950955131,479.359791872623));
#50687=CARTESIAN_POINT('Ctrl Pts',(210.437198595458,-70.645062585471,479.332582761523));
#50688=CARTESIAN_POINT('Ctrl Pts',(210.488635525948,-70.780329866032,479.200142478203));
#50689=CARTESIAN_POINT('Ctrl Pts',(210.596397787298,-71.013440751854,478.920111957033));
#50690=CARTESIAN_POINT('Ctrl Pts',(210.766723027648,-71.293762523166,478.470340135433));
#50691=CARTESIAN_POINT('Ctrl Pts',(210.971444847848,-71.549628732834,477.920756457143));
#50692=CARTESIAN_POINT('Ctrl Pts',(211.214287422258,-71.771639918358,477.257793073053));
#50693=CARTESIAN_POINT('Ctrl Pts',(211.498180471698,-71.942527322346,476.469123872683));
#50694=CARTESIAN_POINT('Ctrl Pts',(211.730850264618,-72.009638215756,475.810711396473));
#50695=CARTESIAN_POINT('Ctrl Pts',(211.866917304058,-72.021141169012,475.421032570143));
#50696=CARTESIAN_POINT('Ctrl Pts',(211.895520581278,-72.022313562161,475.338910192213));
#50697=CARTESIAN_POINT('',(210.277543128129,-70.742002685702,479.379320405933));
#50698=CARTESIAN_POINT('Origin',(211.655917770968,-72.011994055132,481.093613272963));
#50699=CARTESIAN_POINT('Ctrl Pts',(210.277557169171,-70.7420068809479,479.379305544522));
#50700=CARTESIAN_POINT('Ctrl Pts',(210.280160578741,-70.7492044424187,479.371880371481));
#50701=CARTESIAN_POINT('Ctrl Pts',(210.282790072534,-70.7563928376239,479.364380567364));
#50702=CARTESIAN_POINT('Ctrl Pts',(210.285445698698,-70.7635713390691,479.356806032728));
#50703=CARTESIAN_POINT('Ctrl Pts',(210.303010512012,-70.8110513042353,479.306706629199));
#50704=CARTESIAN_POINT('Ctrl Pts',(210.321719670561,-70.8580999963955,479.253334602992));
#50705=CARTESIAN_POINT('Ctrl Pts',(210.34159323712,-70.9045511124946,479.196644783729));
#50706=CARTESIAN_POINT('Ctrl Pts',(210.356825602417,-70.9401542019962,479.153194100979));
#50707=CARTESIAN_POINT('Ctrl Pts',(210.372741792365,-70.9754058614108,479.107795006256));
#50708=CARTESIAN_POINT('Ctrl Pts',(210.389344701098,-71.0102232739627,479.060445491085));
#50709=CARTESIAN_POINT('Ctrl Pts',(210.397959575153,-71.0282892423349,479.035876897935));
#50710=CARTESIAN_POINT('Ctrl Pts',(210.406759745185,-71.0462403635195,479.010780894366));
#50711=CARTESIAN_POINT('Ctrl Pts',(210.415743205009,-71.0640622097134,478.985162468652));
#50712=CARTESIAN_POINT('Ctrl Pts',(210.437592471152,-71.1074078992673,478.922854202955));
#50713=CARTESIAN_POINT('Ctrl Pts',(210.460527104185,-71.1499888075461,478.857452485973));
#50714=CARTESIAN_POINT('Ctrl Pts',(210.484528025454,-71.1916308944509,478.788999974412));
#50715=CARTESIAN_POINT('Ctrl Pts',(210.498241624089,-71.2154242672025,478.749887714571));
#50716=CARTESIAN_POINT('Ctrl Pts',(210.512303025228,-71.2389111258196,478.709780310016));
#50717=CARTESIAN_POINT('Ctrl Pts',(210.526706043544,-71.2620589077047,478.668692955888));
#50718=CARTESIAN_POINT('Ctrl Pts',(210.54338313569,-71.2888614627661,478.621118372854));
#50719=CARTESIAN_POINT('Ctrl Pts',(210.560526992361,-71.3152111239887,478.572222070248));
#50720=CARTESIAN_POINT('Ctrl Pts',(210.578151125547,-71.3410926562255,478.521961253831));
#50721=CARTESIAN_POINT('Ctrl Pts',(210.605101823219,-71.3806705091173,478.445102774968));
#50722=CARTESIAN_POINT('Ctrl Pts',(210.633175694648,-71.4191559802251,478.365053363194));
#50723=CARTESIAN_POINT('Ctrl Pts',(210.662445142328,-71.4564687983787,478.281589220188));
#50724=CARTESIAN_POINT('Ctrl Pts',(210.67139173563,-71.4678739541101,478.256077302406));
#50725=CARTESIAN_POINT('Ctrl Pts',(210.680450001339,-71.479169193652,478.230246415156));
#50726=CARTESIAN_POINT('Ctrl Pts',(210.689621898206,-71.4903512773119,478.204090432413));
#50727=CARTESIAN_POINT('Ctrl Pts',(210.716593016753,-71.5232336034355,478.127175469087));
#50728=CARTESIAN_POINT('Ctrl Pts',(210.744552198908,-71.5551392419009,478.047446978764));
#50729=CARTESIAN_POINT('Ctrl Pts',(210.773572311252,-71.5859845480201,477.964692299568));
#50730=CARTESIAN_POINT('Ctrl Pts',(210.802831346308,-71.6170838036805,477.881256300735));
#50731=CARTESIAN_POINT('Ctrl Pts',(210.833168720309,-71.6471054203407,477.794744452416));
#50732=CARTESIAN_POINT('Ctrl Pts',(210.864674824082,-71.6759139021875,477.704893419951));
#50733=CARTESIAN_POINT('Ctrl Pts',(210.870046833889,-71.6808259486946,477.689573194036));
#50734=CARTESIAN_POINT('Ctrl Pts',(210.875452808655,-71.6857026097514,477.67415592533));
#50735=CARTESIAN_POINT('Ctrl Pts',(210.880893177905,-71.6905430691913,477.658640359874));
#50736=CARTESIAN_POINT('Ctrl Pts',(210.911737968914,-71.7179866034388,477.570673100312));
#50737=CARTESIAN_POINT('Ctrl Pts',(210.943686396808,-71.7442659054198,477.479554290886));
#50738=CARTESIAN_POINT('Ctrl Pts',(210.976804992788,-71.7691988042492,477.385104399128));
#50739=CARTESIAN_POINT('Ctrl Pts',(210.987054560879,-71.7769150566051,477.35587397531));
#50740=CARTESIAN_POINT('Ctrl Pts',(210.997416127991,-71.7845020756729,477.32632473439));
#50741=CARTESIAN_POINT('Ctrl Pts',(211.007891432172,-71.7919537134947,477.296452039278));
#50742=CARTESIAN_POINT('Ctrl Pts',(211.039279596389,-71.8142817745812,477.20694160181));
#50743=CARTESIAN_POINT('Ctrl Pts',(211.071689486874,-71.8353967743902,477.114525462315));
#50744=CARTESIAN_POINT('Ctrl Pts',(211.105177594679,-71.8551008150377,477.019051458798));
#50745=CARTESIAN_POINT('Ctrl Pts',(211.138084368878,-71.8744628052758,476.925234827115));
#50746=CARTESIAN_POINT('Ctrl Pts',(211.172019133444,-71.892457782187,476.828475866872));
#50747=CARTESIAN_POINT('Ctrl Pts',(211.206907722279,-71.9088265655436,476.728987212169));
#50748=CARTESIAN_POINT('Ctrl Pts',(211.233014365774,-71.9210750973934,476.654541242101));
#50749=CARTESIAN_POINT('Ctrl Pts',(211.259654769354,-71.9324134528417,476.578567736639));
#50750=CARTESIAN_POINT('Ctrl Pts',(211.286792129693,-71.9427410029755,476.501172213991));
#50751=CARTESIAN_POINT('Ctrl Pts',(211.312411494309,-71.9524908559146,476.428106002336));
#50752=CARTESIAN_POINT('Ctrl Pts',(211.338473676087,-71.9613399669066,476.353772691105));
#50753=CARTESIAN_POINT('Ctrl Pts',(211.364948044876,-71.9692011295693,476.278260167726));
#50754=CARTESIAN_POINT('Ctrl Pts',(211.403692567548,-71.9807057285056,476.167749632144));
#50755=CARTESIAN_POINT('Ctrl Pts',(211.443318711821,-71.9900966506597,476.054722035542));
#50756=CARTESIAN_POINT('Ctrl Pts',(211.483835022319,-71.9971271824968,475.939162362379));
#50757=CARTESIAN_POINT('Ctrl Pts',(211.524351332817,-72.0041577143339,475.823602689217));
#50758=CARTESIAN_POINT('Ctrl Pts',(211.565758028763,-72.0088279534614,475.705510341515));
#50759=CARTESIAN_POINT('Ctrl Pts',(211.608049442047,-72.0108586572647,475.584910908401));
#50760=CARTESIAN_POINT('Ctrl Pts',(211.62388197629,-72.0116188869426,475.539762389916));
#50761=CARTESIAN_POINT('Ctrl Pts',(211.639838343728,-72.012008864435,475.494262958125));
#50762=CARTESIAN_POINT('Ctrl Pts',(211.655917770953,-72.0120105964115,475.44841530268));
#50763=CARTESIAN_POINT('Origin',(317.344642938098,-69.47200726879,390.467477301753));
#50764=CARTESIAN_POINT('',(220.926808864541,-70.7420844858612,470.816561573067));
#50765=CARTESIAN_POINT('Origin',(219.548450751088,-69.47200726879,469.102280889483));
#50766=CARTESIAN_POINT('',(220.926793321158,-70.742010897009,470.816601139763));
#50767=CARTESIAN_POINT('Origin',(219.548450751088,-69.47200726879,469.102280889483));
#50768=CARTESIAN_POINT('Origin',(219.548426423888,-69.4721780735883,469.102247110923));
#50769=CARTESIAN_POINT('Origin',(219.548450751088,-69.47200726879,469.102280889483));
#50770=CARTESIAN_POINT('Origin',(263.115917770968,-69.47200726879,445.000000551893));
#50771=CARTESIAN_POINT('Ctrl Pts',(220.743942614928,-70.841025529003,470.882368461713));
#50772=CARTESIAN_POINT('Ctrl Pts',(220.766984976348,-70.713370319682,470.948607761433));
#50773=CARTESIAN_POINT('Ctrl Pts',(220.831469127998,-70.4246254674543,471.129903538223));
#50774=CARTESIAN_POINT('Ctrl Pts',(220.971244196048,-70.0353627526102,471.494352564573));
#50775=CARTESIAN_POINT('Ctrl Pts',(221.172069843028,-69.7138478805081,471.964996709473));
#50776=CARTESIAN_POINT('Ctrl Pts',(221.415156299428,-69.5133172296706,472.474231282293));
#50777=CARTESIAN_POINT('Ctrl Pts',(221.617949220798,-69.4612216318851,472.854013581933));
#50778=CARTESIAN_POINT('Ctrl Pts',(221.733039042858,-69.4642140921138,473.056027688663));
#50779=CARTESIAN_POINT('Ctrl Pts',(221.751139833958,-69.4654397984221,473.087490581763));
#50780=CARTESIAN_POINT('Ctrl Pts',(222.160456726778,-70.78217857104,469.976495610993));
#50781=CARTESIAN_POINT('Ctrl Pts',(222.188437764768,-70.65379562633,470.050541672503));
#50782=CARTESIAN_POINT('Ctrl Pts',(222.264991790468,-70.3700937558322,470.250598510653));
#50783=CARTESIAN_POINT('Ctrl Pts',(222.418383534888,-70.0138432466795,470.636006555953));
#50784=CARTESIAN_POINT('Ctrl Pts',(222.618697713718,-69.7486471121804,471.105944703483));
#50785=CARTESIAN_POINT('Ctrl Pts',(222.842402309448,-69.6065541583209,471.587319564183));
#50786=CARTESIAN_POINT('Ctrl Pts',(223.019053538838,-69.5866015108655,471.930604628433));
#50787=CARTESIAN_POINT('Ctrl Pts',(223.117750638108,-69.6011568594972,472.110264950363));
#50788=CARTESIAN_POINT('Ctrl Pts',(223.133244421858,-69.6040467889201,472.138186261513));
#50789=CARTESIAN_POINT('Ctrl Pts',(222.452890157098,-70.1428865776801,468.447972465233));
#50790=CARTESIAN_POINT('Ctrl Pts',(222.505721982168,-69.9491917378316,468.554105655433));
#50791=CARTESIAN_POINT('Ctrl Pts',(222.649435816318,-69.5229124374613,468.840347590763));
#50792=CARTESIAN_POINT('Ctrl Pts',(222.931550749668,-68.9946418506585,469.388700140293));
#50793=CARTESIAN_POINT('Ctrl Pts',(223.288048531598,-68.6097419549078,470.052830454413));
#50794=CARTESIAN_POINT('Ctrl Pts',(223.671268133938,-68.410944976237,470.729926687363));
#50795=CARTESIAN_POINT('Ctrl Pts',(223.962129370818,-68.389326074635,471.212424905133));
#50796=CARTESIAN_POINT('Ctrl Pts',(224.121103779498,-68.41430577095,471.465655686903));
#50797=CARTESIAN_POINT('Ctrl Pts',(224.145979255988,-68.419099312272,471.505032467103));
#50798=CARTESIAN_POINT('Ctrl Pts',(221.415842816088,-69.3721769829706,467.370406754793));
#50799=CARTESIAN_POINT('Ctrl Pts',(221.495982783688,-69.0944600128107,467.510370006663));
#50800=CARTESIAN_POINT('Ctrl Pts',(221.714774494368,-68.478126745993,467.889686180993));
#50801=CARTESIAN_POINT('Ctrl Pts',(222.150306228938,-67.693627670348,468.628519370763));
#50802=CARTESIAN_POINT('Ctrl Pts',(222.709982073808,-67.097079327632,469.545342858623));
#50803=CARTESIAN_POINT('Ctrl Pts',(223.319573019498,-66.766264510463,470.504270304253));
#50804=CARTESIAN_POINT('Ctrl Pts',(223.784776866048,-66.710340497797,471.203911197863));
#50805=CARTESIAN_POINT('Ctrl Pts',(224.038360896088,-66.737284122903,471.574962089193));
#50806=CARTESIAN_POINT('Ctrl Pts',(224.078017229698,-66.742883601444,471.632745269773));
#50807=CARTESIAN_POINT('Ctrl Pts',(220.926793321158,-70.742010897009,470.816601139763));
#50808=CARTESIAN_POINT('Ctrl Pts',(220.954019546588,-70.609423932937,470.892937850223));
#50809=CARTESIAN_POINT('Ctrl Pts',(221.017898643648,-70.3602758137923,471.067167472223));
#50810=CARTESIAN_POINT('Ctrl Pts',(221.140717502368,-70.0432002664185,471.381409203203));
#50811=CARTESIAN_POINT('Ctrl Pts',(221.288915933368,-69.7913397688457,471.732484521923));
#50812=CARTESIAN_POINT('Ctrl Pts',(221.460643994418,-69.6083606197754,472.107646252993));
#50813=CARTESIAN_POINT('Ctrl Pts',(221.65355487452,-69.4970261598067,472.495428146088));
#50814=CARTESIAN_POINT('Ctrl Pts',(221.7939110984,-69.4720061889133,472.755478514282));
#50815=CARTESIAN_POINT('Ctrl Pts',(221.866228108069,-69.4720072829599,472.883816237293));
#50816=CARTESIAN_POINT('Origin',(221.866229658798,-66.93200726879,472.883818989273));
#50817=CARTESIAN_POINT('Origin',(263.115917770968,-66.93200726879,445.000000551893));
#50818=CARTESIAN_POINT('Origin',(317.464909153118,-72.01200726879,396.015965372443));
#50819=CARTESIAN_POINT('Origin',(211.655917770968,-72.01200726879,481.093605606543));
#50820=CARTESIAN_POINT('Origin',(211.655917770968,-72.01200726879,481.093605606543));
#50821=CARTESIAN_POINT('Origin',(305.864311867508,-72.0120072687901,496.460000551893));
#50822=CARTESIAN_POINT('Origin',(227.022312716318,-72.01200726879,496.460000551893));
#50823=CARTESIAN_POINT('Origin',(227.022312716318,-72.01200726879,496.460000551893));
#50824=CARTESIAN_POINT('Ctrl Pts',(300.593104002278,-72.7677512570001,498.460410335103));
#50825=CARTESIAN_POINT('Ctrl Pts',(300.530601966458,-72.8415267130751,498.467865703403));
#50826=CARTESIAN_POINT('Ctrl Pts',(300.228734977818,-73.1792881921421,498.503643117423));
#50827=CARTESIAN_POINT('Ctrl Pts',(299.613647012858,-73.7177818201391,498.573974279533));
#50828=CARTESIAN_POINT('Ctrl Pts',(298.687681543188,-74.2773859034231,498.671516960093));
#50829=CARTESIAN_POINT('Ctrl Pts',(297.629286318018,-74.6941844569291,498.770637036323));
#50830=CARTESIAN_POINT('Ctrl Pts',(296.436962017048,-74.9488215698491,498.864713036083));
#50831=CARTESIAN_POINT('Ctrl Pts',(295.116742985068,-75.0078404229171,498.944324324143));
#50832=CARTESIAN_POINT('Ctrl Pts',(294.096734072578,-74.8793277233351,498.981804574093));
#50833=CARTESIAN_POINT('Ctrl Pts',(293.523716758098,-74.7445966300441,498.992925994703));
#50834=CARTESIAN_POINT('Ctrl Pts',(293.404307436158,-74.7136854275461,498.994784080203));
#50835=CARTESIAN_POINT('Ctrl Pts',(299.502629808648,-72.0150401412131,499.497186230093));
#50836=CARTESIAN_POINT('Ctrl Pts',(299.447350359308,-72.0696574342111,499.498329782803));
#50837=CARTESIAN_POINT('Ctrl Pts',(299.180702325308,-72.3183990485601,499.503396635393));
#50838=CARTESIAN_POINT('Ctrl Pts',(298.640699616528,-72.7034694767341,499.508897695653));
#50839=CARTESIAN_POINT('Ctrl Pts',(297.836986338008,-73.0785538001051,499.502527801293));
#50840=CARTESIAN_POINT('Ctrl Pts',(296.929923102898,-73.3269041512491,499.474828839513));
#50841=CARTESIAN_POINT('Ctrl Pts',(295.922404003468,-73.4353515823531,499.415978915893));
#50842=CARTESIAN_POINT('Ctrl Pts',(294.824652130248,-73.3818065903941,499.313593060243));
#50843=CARTESIAN_POINT('Ctrl Pts',(293.992560697738,-73.2090456373971,499.198969606623));
#50844=CARTESIAN_POINT('Ctrl Pts',(293.531580251618,-73.0666989540421,499.119994613703));
#50845=CARTESIAN_POINT('Ctrl Pts',(293.435818046288,-73.0350067849761,499.102862236873));
#50846=CARTESIAN_POINT('Ctrl Pts',(298.145838415288,-71.0785068454431,499.161577262733));
#50847=CARTESIAN_POINT('Ctrl Pts',(298.105919591678,-71.1136849925871,499.154867854153));
#50848=CARTESIAN_POINT('Ctrl Pts',(297.913011556038,-71.2742945628341,499.121976194783));
#50849=CARTESIAN_POINT('Ctrl Pts',(297.518836716058,-71.5264525149991,499.049965219793));
#50850=CARTESIAN_POINT('Ctrl Pts',(296.922378360898,-71.7799841162821,498.927010516623));
#50851=CARTESIAN_POINT('Ctrl Pts',(296.236766416838,-71.9582914907431,498.767069704883));
#50852=CARTESIAN_POINT('Ctrl Pts',(295.459642360898,-72.0525390598591,498.561581888153));
#50853=CARTESIAN_POINT('Ctrl Pts',(294.593238217878,-72.0476828902761,498.300987152743));
#50854=CARTESIAN_POINT('Ctrl Pts',(293.918525284618,-71.9600636709791,498.068785636793));
#50855=CARTESIAN_POINT('Ctrl Pts',(293.537339696038,-71.8813627885121,497.925749451273));
#50856=CARTESIAN_POINT('Ctrl Pts',(293.457805978338,-71.8636344410641,497.895359301223));
#50857=CARTESIAN_POINT('Ctrl Pts',(297.475709091698,-70.6159509551311,497.689307502413));
#50858=CARTESIAN_POINT('Ctrl Pts',(297.448499980598,-70.6450625854711,497.678719727403));
#50859=CARTESIAN_POINT('Ctrl Pts',(297.316059697278,-70.7803298660321,497.627282796913));
#50860=CARTESIAN_POINT('Ctrl Pts',(297.036029176108,-71.0134407518541,497.519520535563));
#50861=CARTESIAN_POINT('Ctrl Pts',(296.586257354508,-71.2937625231661,497.349195295213));
#50862=CARTESIAN_POINT('Ctrl Pts',(296.036673676218,-71.5496287328341,497.144473475013));
#50863=CARTESIAN_POINT('Ctrl Pts',(295.373710292128,-71.7716399183581,496.901630900603));
#50864=CARTESIAN_POINT('Ctrl Pts',(294.585041091768,-71.9425273223461,496.617737851163));
#50865=CARTESIAN_POINT('Ctrl Pts',(293.926628615548,-72.0096382157561,496.385068058243));
#50866=CARTESIAN_POINT('Ctrl Pts',(293.536949789218,-72.0211411690121,496.249001018803));
#50867=CARTESIAN_POINT('Ctrl Pts',(293.454827411288,-72.0223135621611,496.220397741583));
#50868=CARTESIAN_POINT('Origin',(263.115917770968,-56.01200726879,445.000000551893));
#50869=CARTESIAN_POINT('',(262.871473015597,-53.47200726879,489.709332148996));
#50870=CARTESIAN_POINT('Origin',(263.115917770968,-53.47200726879,445.000000551893));
#50871=CARTESIAN_POINT('Origin',(262.871473014686,-56.01200726879,489.709332315644));
#50872=CARTESIAN_POINT('Origin',(263.115917770968,-53.47200726879,445.000000551893));
#50873=CARTESIAN_POINT('',(263.50896067409,-53.47200726879,483.287981846615));
#50874=CARTESIAN_POINT('Origin',(263.115917770968,-53.47200726879,445.000000551893));
#50875=CARTESIAN_POINT('Origin',(263.115917770968,-56.01200726879,445.000000551893));
#50876=CARTESIAN_POINT('',(263.115917770968,-56.01200726879,480.750000551893));
#50877=CARTESIAN_POINT('',(263.482887849132,-56.01200726879,480.748117047196));
#50878=CARTESIAN_POINT('Origin',(263.115917770968,-56.01200726879,445.000000551893));
#50879=CARTESIAN_POINT('Origin',(263.115917770968,-56.01200726879,445.000000551893));
#50880=CARTESIAN_POINT('Origin',(263.508960688251,-56.01200726879,483.287983226163));
#50881=CARTESIAN_POINT('Origin',(263.115917770968,-86.89200726879,445.000000551893));
#50882=CARTESIAN_POINT('',(263.115917770968,-55.25000726879,480.750000551893));
#50883=CARTESIAN_POINT('Origin',(263.115917770968,-55.25000726879,445.000000551893));
#50884=CARTESIAN_POINT('',(263.115917770968,-86.89200726879,480.750000551893));
#50885=CARTESIAN_POINT('Origin',(263.115917770968,-55.25000726879,445.000000551893));
#50886=CARTESIAN_POINT('',(263.115917770968,-55.25000726879,472.315000551893));
#50887=CARTESIAN_POINT('Origin',(263.115917770968,-55.25000726879,445.000000551893));
#50888=CARTESIAN_POINT('Origin',(263.115917770968,-86.89200726879,445.000000551893));
#50889=CARTESIAN_POINT('',(263.115917770968,-56.01200726879,472.315000551893));
#50890=CARTESIAN_POINT('Origin',(263.115917770968,-56.01200726879,445.000000551893));
#50891=CARTESIAN_POINT('',(263.115917770968,-86.89200726879,472.315000551893));
#50892=CARTESIAN_POINT('Origin',(263.115917770968,-56.01200726879,445.000000551893));
#50893=CARTESIAN_POINT('',(263.115917770968,-56.01200726879,468.435000551893));
#50894=CARTESIAN_POINT('Origin',(263.115917770968,-56.01200726879,445.000000551893));
#50895=CARTESIAN_POINT('Origin',(263.115917770968,-86.89200726879,445.000000551893));
#50896=CARTESIAN_POINT('',(263.115917770968,-36.07200726879,468.435000551893));
#50897=CARTESIAN_POINT('Origin',(263.115917770968,-36.07200726879,445.000000551893));
#50898=CARTESIAN_POINT('',(263.115917770968,-86.89200726879,468.435000551893));
#50899=CARTESIAN_POINT('Origin',(263.115917770968,-36.07200726879,445.000000551893));
#50900=CARTESIAN_POINT('',(263.115917770968,-36.07200726879,460.000000551893));
#50901=CARTESIAN_POINT('Origin',(263.115917770968,-36.07200726879,445.000000551893));
#50902=CARTESIAN_POINT('Origin',(263.115917770968,-86.89200726879,445.000000551893));
#50903=CARTESIAN_POINT('',(263.115917770968,-84.47200726879,460.000000551893));
#50904=CARTESIAN_POINT('Origin',(263.115917770968,-84.47200726879,445.000000551893));
#50905=CARTESIAN_POINT('',(263.115917770968,-86.89200726879,460.000000551893));
#50906=CARTESIAN_POINT('Origin',(263.115917770968,-84.47200726879,445.000000551893));
#50907=CARTESIAN_POINT('',(263.115917770968,-84.47200726879,468.435000551893));
#50908=CARTESIAN_POINT('Origin',(263.115917770968,-84.47200726879,445.000000551893));
#50909=CARTESIAN_POINT('Origin',(263.115917770968,-86.89200726879,445.000000551893));
#50910=CARTESIAN_POINT('',(263.115917770968,-76.33200726879,468.435000551893));
#50911=CARTESIAN_POINT('Origin',(263.115917770968,-76.33200726879,445.000000551893));
#50912=CARTESIAN_POINT('',(263.115917770968,-86.89200726879,468.435000551893));
#50913=CARTESIAN_POINT('Origin',(263.115917770968,-76.33200726879,445.000000551893));
#50914=CARTESIAN_POINT('',(263.115917770968,-76.33200726879,472.315000551893));
#50915=CARTESIAN_POINT('Origin',(263.115917770968,-76.33200726879,445.000000551893));
#50916=CARTESIAN_POINT('Origin',(263.115917770968,-86.89200726879,445.000000551893));
#50917=CARTESIAN_POINT('',(263.115917770968,-77.0940072687901,472.315000551893));
#50918=CARTESIAN_POINT('Origin',(263.115917770968,-77.09400726879,445.000000551893));
#50919=CARTESIAN_POINT('',(263.115917770968,-86.89200726879,472.315000551893));
#50920=CARTESIAN_POINT('Origin',(263.115917770968,-77.09400726879,445.000000551893));
#50921=CARTESIAN_POINT('',(263.115917770968,-77.09400726879,480.750000551893));
#50922=CARTESIAN_POINT('Origin',(263.115917770968,-77.09400726879,445.000000551893));
#50923=CARTESIAN_POINT('Origin',(263.115917770968,-85.47200726879,445.000000551893));
#50924=CARTESIAN_POINT('',(263.115917770968,-81.66200726879,480.750000551893));
#50925=CARTESIAN_POINT('Origin',(263.115917770968,-81.66200726879,445.000000551893));
#50926=CARTESIAN_POINT('',(263.115917770968,-85.47200726879,480.750000551893));
#50927=CARTESIAN_POINT('Origin',(263.115917770968,-81.66200726879,445.000000551893));
#50928=CARTESIAN_POINT('',(293.115917770968,-81.66200726879,403.500000551893));
#50929=CARTESIAN_POINT('',(304.615917770968,-81.66200726879,415.000000551893));
#50930=CARTESIAN_POINT('Origin',(304.615917770968,-81.66200726879,403.500000551893));
#50931=CARTESIAN_POINT('',(304.615917770968,-81.66200726879,475.000000551893));
#50932=CARTESIAN_POINT('',(304.615917770968,-81.66200726879,415.000000551893));
#50933=CARTESIAN_POINT('',(293.115917770968,-81.66200726879,486.500000551893));
#50934=CARTESIAN_POINT('Origin',(304.615917770968,-81.6620072687901,486.500000551893));
#50935=CARTESIAN_POINT('',(233.115917770968,-81.66200726879,486.500000551893));
#50936=CARTESIAN_POINT('',(293.115917770968,-81.66200726879,486.500000551893));
#50937=CARTESIAN_POINT('',(221.615917770968,-81.66200726879,475.000000551893));
#50938=CARTESIAN_POINT('Origin',(221.615917770968,-81.66200726879,486.500000551893));
#50939=CARTESIAN_POINT('',(221.615917770968,-81.6620072687899,415.000000551893));
#50940=CARTESIAN_POINT('',(221.615917770968,-81.66200726879,475.000000551893));
#50941=CARTESIAN_POINT('',(233.115917770968,-81.6620072687899,403.500000551893));
#50942=CARTESIAN_POINT('Origin',(221.615917770968,-81.6620072687899,403.500000551893));
#50943=CARTESIAN_POINT('',(233.115917770968,-81.6620072687899,403.500000551893));
#50944=CARTESIAN_POINT('Origin',(304.615917770968,-85.47200726879,403.500000551893));
#50945=CARTESIAN_POINT('',(304.615917770968,-85.47200726879,415.000000551893));
#50946=CARTESIAN_POINT('',(293.115917770968,-85.47200726879,403.500000551893));
#50947=CARTESIAN_POINT('Origin',(233.115917770968,-85.4720072687899,403.500000551893));
#50948=CARTESIAN_POINT('',(233.115917770968,-85.4720072687899,403.500000551893));
#50949=CARTESIAN_POINT('Origin',(221.615917770968,-85.4720072687899,403.500000551893));
#50950=CARTESIAN_POINT('',(221.615917770968,-85.47200726879,415.000000551893));
#50951=CARTESIAN_POINT('Origin',(221.615917770968,-85.47200726879,475.000000551893));
#50952=CARTESIAN_POINT('',(221.615917770968,-85.47200726879,475.000000551893));
#50953=CARTESIAN_POINT('Origin',(221.615917770968,-85.47200726879,486.500000551893));
#50954=CARTESIAN_POINT('',(233.115917770968,-85.47200726879,486.500000551893));
#50955=CARTESIAN_POINT('Origin',(293.115917770968,-85.4720072687901,486.500000551893));
#50956=CARTESIAN_POINT('',(293.115917770968,-85.4720072687901,486.500000551893));
#50957=CARTESIAN_POINT('Origin',(304.615917770968,-85.4720072687901,486.500000551893));
#50958=CARTESIAN_POINT('',(304.615917770968,-85.4720072687901,475.000000551893));
#50959=CARTESIAN_POINT('Origin',(304.615917770968,-85.47200726879,415.000000551893));
#61752=UNCERTAINTY_MEASURE_WITH_UNIT(LENGTH_MEASURE(0.01),#61812,
'DISTANCE_ACCURACY_VALUE',
'Maximum model space distance between geometric entities at asserted c
onnectivities');
#61780=UNCERTAINTY_MEASURE_WITH_UNIT(LENGTH_MEASURE(0.01),#61812,
'DISTANCE_ACCURACY_VALUE',
'Maximum model space distance between geometric entities at asserted c
onnectivities');
#61783=(
GEOMETRIC_REPRESENTATION_CONTEXT(3)
GLOBAL_UNCERTAINTY_ASSIGNED_CONTEXT((#61752))
GLOBAL_UNIT_ASSIGNED_CONTEXT((#61812,#61814,#61815))
REPRESENTATION_CONTEXT('','3D')
);
#61811=(
GEOMETRIC_REPRESENTATION_CONTEXT(3)
GLOBAL_UNCERTAINTY_ASSIGNED_CONTEXT((#61780))
GLOBAL_UNIT_ASSIGNED_CONTEXT((#61812,#61814,#61815))
REPRESENTATION_CONTEXT('','3D')
);
#61812=(
LENGTH_UNIT()
NAMED_UNIT(*)
SI_UNIT(.MILLI.,.METRE.)
);
#61814=(
NAMED_UNIT(*)
PLANE_ANGLE_UNIT()
SI_UNIT($,.RADIAN.)
);
#61815=(
NAMED_UNIT(*)
SI_UNIT($,.STERADIAN.)
SOLID_ANGLE_UNIT()
);
#61818=SHAPE_DEFINITION_REPRESENTATION(#61848,#61970);
#61848=PRODUCT_DEFINITION_SHAPE('',$,#62001);
#61970=SHAPE_REPRESENTATION('',(#34153),#61783);
#61998=PRODUCT_DEFINITION_CONTEXT('part definition',#62090,'design');
#62001=PRODUCT_DEFINITION('Shaft Bearing Flange Units',
'Shaft Bearing Flange Units',#62031,#61998);
#62031=PRODUCT_DEFINITION_FORMATION('',$,#62094);
#62090=APPLICATION_CONTEXT('Managed model based 3d engineering');
#62091=PRODUCT_CONTEXT('part definition',#62090,'mechanical');
#62094=PRODUCT('Shaft Bearing Flange Units',
'Shaft Bearing Flange Units',$,(#62091));
#62150=COLOUR_RGB('Grey',0.48,0.52,0.57);
#62151=FILL_AREA_STYLE_COLOUR('',#62150);
#62152=FILL_AREA_STYLE('',(#62151));
#62153=SURFACE_STYLE_FILL_AREA(#62152);
#62154=SURFACE_SIDE_STYLE('',(#62153));
#62155=SURFACE_STYLE_USAGE(.BOTH.,#62154);
#62156=PRESENTATION_STYLE_ASSIGNMENT((#62155));
ENDSEC;
END-ISO-10303-21;
